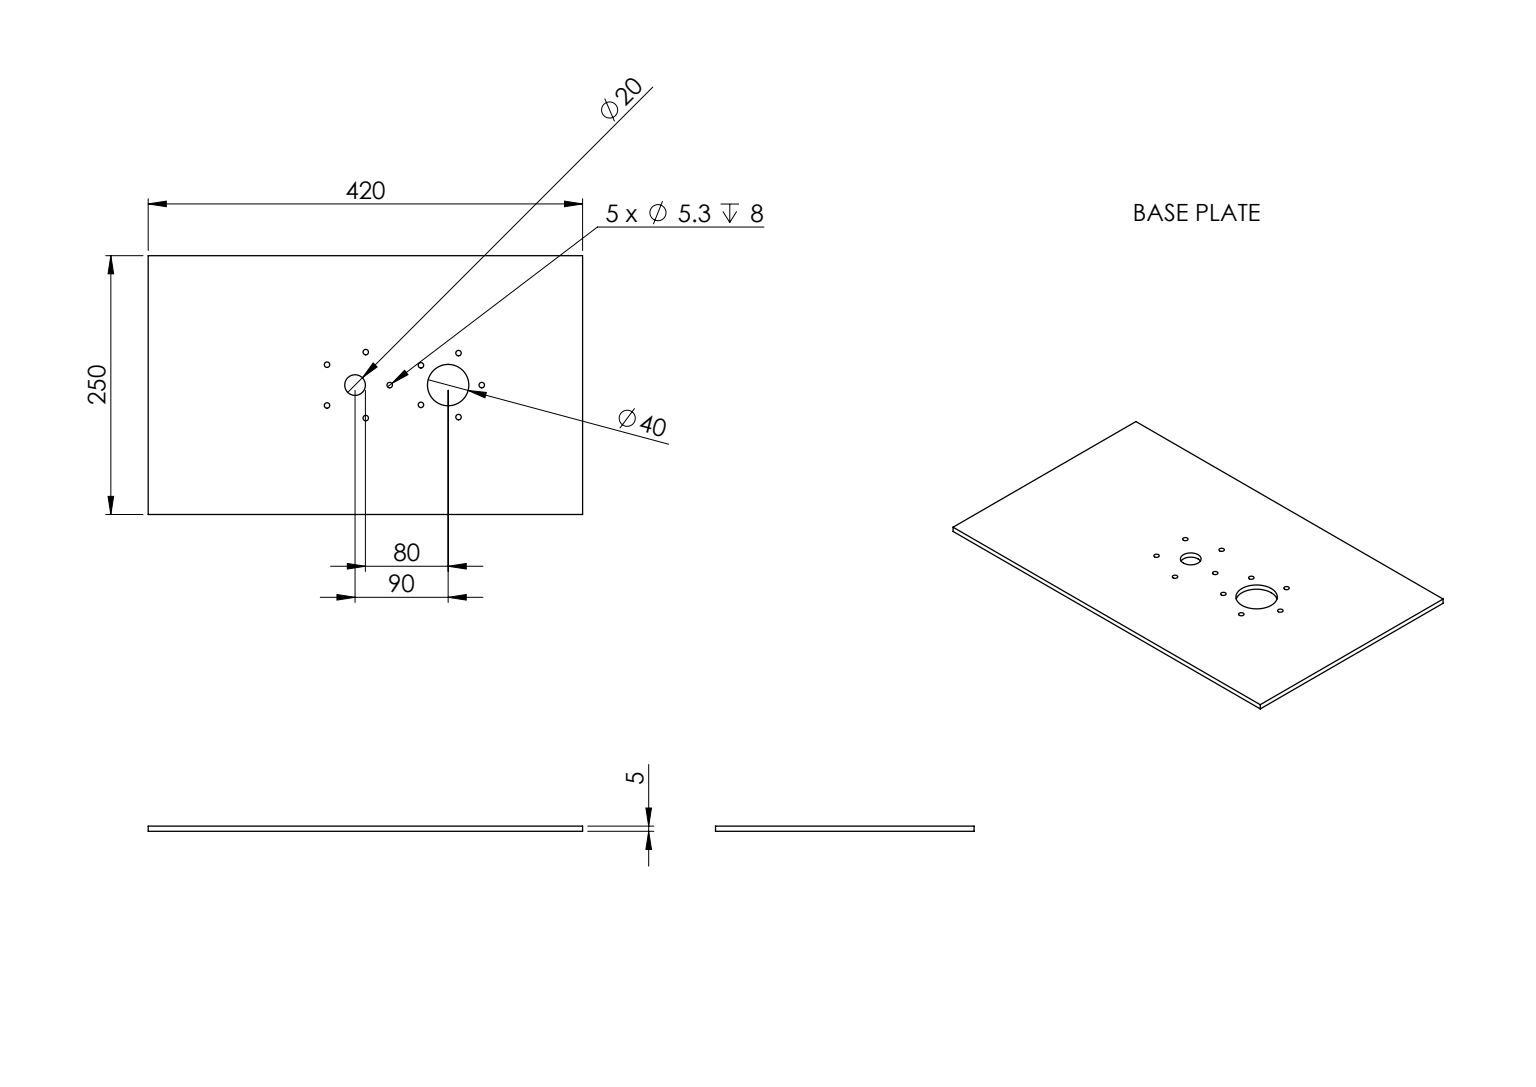
ISO-10303-21;
HEADER;
FILE_DESCRIPTION (('STEP AP214'),
    '1' );
FILE_NAME ('base plate.step',
    '2026-10-24T07:08:27',
    ( '' ),
    ( '' ),
    'SwSTEP 2.0',
    'SolidWorks 2026',
    '' );
FILE_SCHEMA (( 'AUTOMOTIVE_DESIGN' ));
ENDSEC;

DATA;
#6=VERTEX_POINT ( 'NONE', #17079 ) ;
#11=CARTESIAN_POINT ( 'NONE',  ( -79.64793068852898728, -30.00000000000000000, -31.86039329588756530 ) ) ;
#15=FACE_BOUND ( 'NONE', #1592, .T. ) ;
#41=EDGE_CURVE ( 'NONE', #17767, #6918, #12253, .T. ) ;
#44=EDGE_CURVE ( 'NONE', #931, #15024, #4657, .T. ) ;
#71=EDGE_CURVE ( 'NONE', #17356, #16127, #6478, .T. ) ;
#87=FACE_OUTER_BOUND ( 'NONE', #3507, .T. ) ;
#114=VERTEX_POINT ( 'NONE', #13345 ) ;
#120=CARTESIAN_POINT ( 'NONE',  ( -117.1020693116506379, -30.00000000000000000, -19.69080595179801207 ) ) ;
#126=COLOUR_RGB ( '',0.8941176470588234615, 0.8941176470588234615, 0.8941176470588234615 ) ;
#138=FACE_OUTER_BOUND ( 'NONE', #567, .T. ) ;
#139=VERTEX_POINT ( 'NONE', #10380 ) ;
#143=CARTESIAN_POINT ( 'NONE',  ( 0.000000000000000000, -34.99999999999999289, 20.00000000000000000 ) ) ;
#162=EDGE_CURVE ( 'NONE', #3115, #10632, #18771, .T. ) ;
#174=EDGE_CURVE ( 'NONE', #11247, #17285, #17354, .T. ) ;
#227=DIRECTION ( 'NONE',  ( -0.000000000000000000, 1.000000000000000000, -0.000000000000000000 ) ) ;
#242=CARTESIAN_POINT ( 'NONE',  ( 10.04305231718605285, -30.00000000000000000, -30.90933677959240811 ) ) ;
#257=DIRECTION ( 'NONE',  ( -0.000000000000000000, -1.000000000000000000, -0.000000000000000000 ) ) ;
#303=EDGE_CURVE ( 'NONE', #6749, #12292, #6178, .T. ) ;
#306=LINE ( 'NONE', #5042, #9675 ) ;
#312=ORIENTED_EDGE ( 'NONE', *, *, #6097, .T. ) ;
#348=EDGE_LOOP ( 'NONE', ( #7542, #2578 ) ) ;
#362=LINE ( 'NONE', #1882, #10479 ) ;
#365=DIRECTION ( 'NONE',  ( 2.220446049250313081E-16, 0.000000000000000000, 1.000000000000000000 ) ) ;
#372=EDGE_CURVE ( 'NONE', #3496, #11369, #16387, .T. ) ;
#379=EDGE_CURVE ( 'NONE', #3115, #12051, #15919, .T. ) ;
#386=VECTOR ( 'NONE', #8852, 1000.000000000000000 ) ;
#389=CARTESIAN_POINT ( 'NONE',  ( 10.04305231718605285, -26.50000000000000000, -30.90933677959240811 ) ) ;
#398=FILL_AREA_STYLE_COLOUR ( '', #126 ) ;
#409=CYLINDRICAL_SURFACE ( 'NONE', #7915, 2.649999999999995914 ) ;
#421=VERTEX_POINT ( 'NONE', #1046 ) ;
#422=ORIENTED_EDGE ( 'NONE', *, *, #16105, .T. ) ;
#425=DIRECTION ( 'NONE',  ( 0.000000000000000000, 1.000000000000000000, 0.000000000000000000 ) ) ;
#460=CARTESIAN_POINT ( 'NONE',  ( 10.04305231718579705, -30.00000000000000000, 33.55933677959249195 ) ) ;
#481=CARTESIAN_POINT ( 'NONE',  ( -79.64793068852898728, -30.00000000000000000, -31.86039329588756530 ) ) ;
#495=ORIENTED_EDGE ( 'NONE', *, *, #4462, .F. ) ;
#518=EDGE_CURVE ( 'NONE', #10933, #833, #10392, .T. ) ;
#526=ORIENTED_EDGE ( 'NONE', *, *, #16492, .F. ) ;
#533=CARTESIAN_POINT ( 'NONE',  ( 129.9999999999999432, -34.99999999999999289, -125.0000000000000000 ) ) ;
#543=DIRECTION ( 'NONE',  ( 0.000000000000000000, 0.000000000000000000, -1.000000000000000000 ) ) ;
#546=ORIENTED_EDGE ( 'NONE', *, *, #4687, .T. ) ;
#567=EDGE_LOOP ( 'NONE', ( #6055, #18455, #17783, #6474 ) ) ;
#578=EDGE_CURVE ( 'NONE', #13109, #8902, #3719, .T. ) ;
#589=DIRECTION ( 'NONE',  ( 1.000000000000000000, 0.000000000000000000, 0.000000000000000000 ) ) ;
#591=ORIENTED_EDGE ( 'NONE', *, *, #16105, .F. ) ;
#600=CARTESIAN_POINT ( 'NONE',  ( -56.50000000009000445, -34.99999999999999289, 3.817814120399276590E-13 ) ) ;
#672=FACE_OUTER_BOUND ( 'NONE', #6327, .T. ) ;
#682=PRESENTATION_STYLE_ASSIGNMENT (( #9797 ) ) ;
#690=ORIENTED_EDGE ( 'NONE', *, *, #12876, .F. ) ;
#705=EDGE_CURVE ( 'NONE', #15024, #931, #15786, .T. ) ;
#720=CARTESIAN_POINT ( 'NONE',  ( 0.000000000000000000, -34.99999999999999289, 0.000000000000000000 ) ) ;
#766=ORIENTED_EDGE ( 'NONE', *, *, #14475, .F. ) ;
#768=ORIENTED_EDGE ( 'NONE', *, *, #17161, .T. ) ;
#801=ORIENTED_EDGE ( 'NONE', *, *, #4462, .T. ) ;
#809=CIRCLE ( 'NONE', #5971, 2.649999999999999467 ) ;
#813=ORIENTED_EDGE ( 'NONE', *, *, #41, .F. ) ;
#814=CIRCLE ( 'NONE', #9625, 10.00000000000000888 ) ;
#818=FACE_BOUND ( 'NONE', #15309, .T. ) ;
#833=VERTEX_POINT ( 'NONE', #8602 ) ;
#834=ORIENTED_EDGE ( 'NONE', *, *, #10294, .F. ) ;
#842=CARTESIAN_POINT ( 'NONE',  ( -290.0000000000001137, -34.99999999999999289, -125.0000000000000000 ) ) ;
#884=ORIENTED_EDGE ( 'NONE', *, *, #8191, .T. ) ;
#891=VECTOR ( 'NONE', #1458, 1000.000000000000000 ) ;
#917=EDGE_CURVE ( 'NONE', #6918, #17767, #10543, .T. ) ;
#931=VERTEX_POINT ( 'NONE', #2514 ) ;
#992=ORIENTED_EDGE ( 'NONE', *, *, #12234, .T. ) ;
#1000=ORIENTED_EDGE ( 'NONE', *, *, #7256, .T. ) ;
#1005=DIRECTION ( 'NONE',  ( 0.000000000000000000, 0.000000000000000000, 1.000000000000000000 ) ) ;
#1046=CARTESIAN_POINT ( 'NONE',  ( -79.64793068852927149, -34.99999999999999289, 29.21039329588765554 ) ) ;
#1051=CARTESIAN_POINT ( 'NONE',  ( -117.1020693116508085, -34.99999999999999289, 19.69080595179778115 ) ) ;
#1087=CARTESIAN_POINT ( 'NONE',  ( -90.00000000009001155, -34.99999999999999289, -1.301042606982605321E-15 ) ) ;
#1117=ORIENTED_EDGE ( 'NONE', *, *, #2996, .T. ) ;
#1126=EDGE_LOOP ( 'NONE', ( #813, #5939 ) ) ;
#1159=CARTESIAN_POINT ( 'NONE',  ( -26.29305231718568336, -34.99999999999999289, -19.10302069950552095 ) ) ;
#1167=DIRECTION ( 'NONE',  ( 0.000000000000000000, 1.000000000000000000, 0.000000000000000000 ) ) ;
#1245=AXIS2_PLACEMENT_3D ( 'NONE', #17658, #4603, #10410 ) ;
#1248=ORIENTED_EDGE ( 'NONE', *, *, #16015, .T. ) ;
#1296=EDGE_CURVE ( 'NONE', #114, #9433, #4484, .T. ) ;
#1299=CARTESIAN_POINT ( 'NONE',  ( -26.29305231718584324, -26.50000000000000000, 19.10302069950530779 ) ) ;
#1300=ORIENTED_EDGE ( 'NONE', *, *, #11741, .F. ) ;
#1311=CARTESIAN_POINT ( 'NONE',  ( -117.1020693116506379, -30.00000000000000000, -19.69080595179801207 ) ) ;
#1319=CARTESIAN_POINT ( 'NONE',  ( -79.64793068852898728, -30.00000000000000000, -29.21039329588757383 ) ) ;
#1328=EDGE_CURVE ( 'NONE', #10185, #18475, #2082, .T. ) ;
#1405=ORIENTED_EDGE ( 'NONE', *, *, #12009, .T. ) ;
#1414=DIRECTION ( 'NONE',  ( 0.000000000000000000, 0.000000000000000000, 1.000000000000000000 ) ) ;
#1447=ADVANCED_FACE ( 'NONE', ( #16139 ), #17217, .F. ) ;
#1457=AXIS2_PLACEMENT_3D ( 'NONE', #120, #5912, #4495 ) ;
#1458=DIRECTION ( 'NONE',  ( -0.000000000000000000, -1.000000000000000000, -0.000000000000000000 ) ) ;
#1470=VECTOR ( 'NONE', #589, 1000.000000000000000 ) ;
#1476=FACE_OUTER_BOUND ( 'NONE', #11507, .T. ) ;
#1494=VECTOR ( 'NONE', #7308, 1000.000000000000000 ) ;
#1513=DIRECTION ( 'NONE',  ( -0.000000000000000000, 1.000000000000000000, -0.000000000000000000 ) ) ;
#1525=DIRECTION ( 'NONE',  ( 0.000000000000000000, -0.000000000000000000, 1.000000000000000000 ) ) ;
#1567=VERTEX_POINT ( 'NONE', #16419 ) ;
#1574=ORIENTED_EDGE ( 'NONE', *, *, #6302, .T. ) ;
#1583=CARTESIAN_POINT ( 'NONE',  ( -26.29305231718568336, -26.50000000000000000, -16.45302069950552237 ) ) ;
#1584=AXIS2_PLACEMENT_3D ( 'NONE', #11711, #17616, #5719 ) ;
#1592=EDGE_LOOP ( 'NONE', ( #11082, #13432 ) ) ;
#1593=ORIENTED_EDGE ( 'NONE', *, *, #16015, .F. ) ;
#1597=ORIENTED_EDGE ( 'NONE', *, *, #705, .F. ) ;
#1647=CARTESIAN_POINT ( 'NONE',  ( -290.0000000000001137, -34.99999999999999289, -125.0000000000000000 ) ) ;
#1654=EDGE_LOOP ( 'NONE', ( #3997, #6945 ) ) ;
#1700=DIRECTION ( 'NONE',  ( 0.000000000000000000, 1.000000000000000000, 0.000000000000000000 ) ) ;
#1701=ORIENTED_EDGE ( 'NONE', *, *, #15947, .F. ) ;
#1743=DIRECTION ( 'NONE',  ( -0.000000000000000000, -1.000000000000000000, -0.000000000000000000 ) ) ;
#1773=ORIENTED_EDGE ( 'NONE', *, *, #3966, .T. ) ;
#1779=EDGE_LOOP ( 'NONE', ( #16032, #2338, #6206, #546 ) ) ;
#1785=CYLINDRICAL_SURFACE ( 'NONE', #8196, 2.649999999999992806 ) ;
#1833=EDGE_LOOP ( 'NONE', ( #14175, #1300 ) ) ;
#1852=VECTOR ( 'NONE', #18637, 1000.000000000000000 ) ;
#1882=CARTESIAN_POINT ( 'NONE',  ( 130.0000000000000000, -34.99999999999999289, 125.0000000000000000 ) ) ;
#1910=FACE_OUTER_BOUND ( 'NONE', #10213, .T. ) ;
#1919=ADVANCED_FACE ( 'NONE', ( #10204 ), #2787, .F. ) ;
#1976=FACE_OUTER_BOUND ( 'NONE', #7216, .T. ) ;
#1988=DIRECTION ( 'NONE',  ( -0.000000000000000000, -1.000000000000000000, -0.000000000000000000 ) ) ;
#2004=DIRECTION ( 'NONE',  ( -0.000000000000000000, 1.000000000000000000, -0.000000000000000000 ) ) ;
#2019=EDGE_CURVE ( 'NONE', #5476, #6010, #306, .T. ) ;
#2034=LINE ( 'NONE', #6412, #15369 ) ;
#2063=DIRECTION ( 'NONE',  ( 0.000000000000000000, 0.000000000000000000, 1.000000000000000000 ) ) ;
#2079=ADVANCED_FACE ( 'NONE', ( #3250 ), #13448, .F. ) ;
#2082=LINE ( 'NONE', #6544, #18168 ) ;
#2096=DIRECTION ( 'NONE',  ( 0.000000000000000000, 0.000000000000000000, 1.000000000000000000 ) ) ;
#2099=ADVANCED_FACE ( 'NONE', ( #1910 ), #13533, .F. ) ;
#2102=DIRECTION ( 'NONE',  ( -0.000000000000000000, 1.000000000000000000, -0.000000000000000000 ) ) ;
#2142=DIRECTION ( 'NONE',  ( -0.000000000000000000, 1.000000000000000000, -0.000000000000000000 ) ) ;
#2144=FACE_BOUND ( 'NONE', #18626, .T. ) ;
#2188=DIRECTION ( 'NONE',  ( -0.000000000000000000, 1.000000000000000000, -0.000000000000000000 ) ) ;
#2232=ORIENTED_EDGE ( 'NONE', *, *, #12399, .T. ) ;
#2246=( GEOMETRIC_REPRESENTATION_CONTEXT ( 3 ) GLOBAL_UNCERTAINTY_ASSIGNED_CONTEXT ( ( #14139 ) ) GLOBAL_UNIT_ASSIGNED_CONTEXT ( ( #8004, #17231, #15165 ) ) REPRESENTATION_CONTEXT ( 'NONE', 'WORKASPACE' ) );
#2260=VERTEX_POINT ( 'NONE', #16093 ) ;
#2267=VERTEX_POINT ( 'NONE', #14659 ) ;
#2289=EDGE_CURVE ( 'NONE', #10632, #8217, #5434, .T. ) ;
#2299=CARTESIAN_POINT ( 'NONE',  ( -26.29305231718568336, -30.00000000000000000, -16.45302069950552237 ) ) ;
#2307=EDGE_LOOP ( 'NONE', ( #14097, #884, #7375, #8235 ) ) ;
#2310=ORIENTED_EDGE ( 'NONE', *, *, #9236, .T. ) ;
#2316=ORIENTED_EDGE ( 'NONE', *, *, #12234, .F. ) ;
#2338=ORIENTED_EDGE ( 'NONE', *, *, #11370, .F. ) ;
#2339=EDGE_LOOP ( 'NONE', ( #17775, #17142 ) ) ;
#2344=VECTOR ( 'NONE', #9583, 1000.000000000000000 ) ;
#2404=EDGE_LOOP ( 'NONE', ( #3864, #2415 ) ) ;
#2415=ORIENTED_EDGE ( 'NONE', *, *, #303, .F. ) ;
#2422=VERTEX_POINT ( 'NONE', #17894 ) ;
#2494=ADVANCED_FACE ( 'NONE', ( #11888 ), #13334, .F. ) ;
#2497=CARTESIAN_POINT ( 'NONE',  ( -290.0000000000001137, -30.00000000000000000, -125.0000000000000000 ) ) ;
#2499=CYLINDRICAL_SURFACE ( 'NONE', #10518, 2.649999999999995914 ) ;
#2514=CARTESIAN_POINT ( 'NONE',  ( -26.29305231718584324, -34.99999999999999289, 16.45302069950530566 ) ) ;
#2578=ORIENTED_EDGE ( 'NONE', *, *, #11344, .F. ) ;
#2592=CARTESIAN_POINT ( 'NONE',  ( 0.000000000000000000, -30.00000000000000000, 0.000000000000000000 ) ) ;
#2593=CARTESIAN_POINT ( 'NONE',  ( 32.50000000000000000, -34.99999999999999289, 3.680389326632394941E-13 ) ) ;
#2626=DIRECTION ( 'NONE',  ( 0.000000000000000000, 1.000000000000000000, 0.000000000000000000 ) ) ;
#2633=AXIS2_PLACEMENT_3D ( 'NONE', #6245, #17768, #15017 ) ;
#2671=LINE ( 'NONE', #10001, #13888 ) ;
#2678=CARTESIAN_POINT ( 'NONE',  ( -90.00000000009001155, -29.99899999999999878, -1.301042606982605321E-15 ) ) ;
#2679=VECTOR ( 'NONE', #12131, 1000.000000000000000 ) ;
#2705=PRODUCT_CONTEXT ( 'NONE', #4283, 'mechanical' ) ;
#2757=DIRECTION ( 'NONE',  ( 0.000000000000000000, 0.000000000000000000, 1.000000000000000000 ) ) ;
#2770=DIRECTION ( 'NONE',  ( 0.000000000000000000, 1.000000000000000000, 0.000000000000000000 ) ) ;
#2773=STYLED_ITEM('',(#18855),#10108);
#2783=DIRECTION ( 'NONE',  ( -1.000000000000000000, 0.000000000000000000, -0.000000000000000000 ) ) ;
#2787=CYLINDRICAL_SURFACE ( 'NONE', #1457, 2.649999999999992806 ) ;
#2827=EDGE_CURVE ( 'NONE', #16722, #5310, #4082, .T. ) ;
#2846=ADVANCED_FACE ( 'NONE', ( #17872 ), #16535, .F. ) ;
#2854=CARTESIAN_POINT ( 'NONE',  ( -117.1020693116508085, -30.00000000000000000, 22.34080595179776907 ) ) ;
#2864=CARTESIAN_POINT ( 'NONE',  ( 2.449293598294706513E-15, -34.99999999999999289, -20.00000000000000000 ) ) ;
#2868=CARTESIAN_POINT ( 'NONE',  ( 129.9999999999999432, -34.99999999999999289, -125.0000000000000000 ) ) ;
#2885=DIRECTION ( 'NONE',  ( -0.000000000000000000, 1.000000000000000000, -0.000000000000000000 ) ) ;
#2888=ORIENTED_EDGE ( 'NONE', *, *, #17161, .F. ) ;
#2954=EDGE_CURVE ( 'NONE', #3496, #10145, #7497, .T. ) ;
#2979=CIRCLE ( 'NONE', #14535, 2.649999999999995914 ) ;
#2996=EDGE_CURVE ( 'NONE', #15825, #6010, #809, .T. ) ;
#3009=CYLINDRICAL_SURFACE ( 'NONE', #15827, 2.649999999999999467 ) ;
#3019=CARTESIAN_POINT ( 'NONE',  ( 10.04305231718579705, -26.50000000000000000, 28.25933677959249835 ) ) ;
#3089=DIRECTION ( 'NONE',  ( 0.000000000000000000, 0.000000000000000000, 1.000000000000000000 ) ) ;
#3115=VERTEX_POINT ( 'NONE', #3969 ) ;
#3156=DIRECTION ( 'NONE',  ( -0.000000000000000000, 1.000000000000000000, -0.000000000000000000 ) ) ;
#3161=( GEOMETRIC_REPRESENTATION_CONTEXT ( 3 ) GLOBAL_UNCERTAINTY_ASSIGNED_CONTEXT ( ( #15290 ) ) GLOBAL_UNIT_ASSIGNED_CONTEXT ( ( #14683, #18007, #11919 ) ) REPRESENTATION_CONTEXT ( 'NONE', 'WORKASPACE' ) );
#3175=CARTESIAN_POINT ( 'NONE',  ( -56.50000000009000445, -30.00000000000000000, 3.817814120399276590E-13 ) ) ;
#3197=CARTESIAN_POINT ( 'NONE',  ( -117.1020693116506379, -30.00000000000000000, -22.34080595179799644 ) ) ;
#3218=VECTOR ( 'NONE', #2004, 1000.000000000000000 ) ;
#3222=ORIENTED_EDGE ( 'NONE', *, *, #2827, .T. ) ;
#3230=DIRECTION ( 'NONE',  ( 0.000000000000000000, 0.000000000000000000, 1.000000000000000000 ) ) ;
#3233=FACE_BOUND ( 'NONE', #18034, .T. ) ;
#3237=ORIENTED_EDGE ( 'NONE', *, *, #518, .T. ) ;
#3250=FACE_OUTER_BOUND ( 'NONE', #18743, .T. ) ;
#3293=PRODUCT ( 'base plate', 'base plate', '', ( #2705 ) ) ;
#3320=AXIS2_PLACEMENT_3D ( 'NONE', #12306, #11167, #13832 ) ;
#3345=CARTESIAN_POINT ( 'NONE',  ( 32.50000000000000000, -26.50000000000000000, 2.650000000000367617 ) ) ;
#3388=CYLINDRICAL_SURFACE ( 'NONE', #15829, 2.649999999999999467 ) ;
#3415=CYLINDRICAL_SURFACE ( 'NONE', #15730, 2.649999999999992806 ) ;
#3430=DIRECTION ( 'NONE',  ( 0.000000000000000000, 0.000000000000000000, 1.000000000000000000 ) ) ;
#3433=EDGE_CURVE ( 'NONE', #12463, #15108, #11438, .T. ) ;
#3451=ORIENTED_EDGE ( 'NONE', *, *, #4742, .F. ) ;
#3461=DIRECTION ( 'NONE',  ( -0.000000000000000000, 1.000000000000000000, -0.000000000000000000 ) ) ;
#3465=CYLINDRICAL_SURFACE ( 'NONE', #14086, 2.649999999999992806 ) ;
#3490=CARTESIAN_POINT ( 'NONE',  ( -90.00000000009001155, -29.99899999999999878, -1.301042606982605321E-15 ) ) ;
#3496=VERTEX_POINT ( 'NONE', #18587 ) ;
#3507=EDGE_LOOP ( 'NONE', ( #14888, #591, #4877, #1000 ) ) ;
#3509=DIRECTION ( 'NONE',  ( -0.000000000000000000, 1.000000000000000000, -0.000000000000000000 ) ) ;
#3513=ADVANCED_FACE ( 'NONE', ( #9908 ), #15727, .F. ) ;
#3530=AXIS2_PLACEMENT_3D ( 'NONE', #15724, #12775, #17155 ) ;
#3559=AXIS2_PLACEMENT_3D ( 'NONE', #6389, #10947, #13724 ) ;
#3582=AXIS2_PLACEMENT_3D ( 'NONE', #8174, #9587, #15407 ) ;
#3584=FACE_OUTER_BOUND ( 'NONE', #16769, .T. ) ;
#3589=VERTEX_POINT ( 'NONE', #2864 ) ;
#3611=CARTESIAN_POINT ( 'NONE',  ( -79.64793068852898728, -30.00000000000000000, -29.21039329588758093 ) ) ;
#3659=VERTEX_POINT ( 'NONE', #6466 ) ;
#3679=EDGE_LOOP ( 'NONE', ( #8260, #18538, #18212, #10633 ) ) ;
#3692=DIRECTION ( 'NONE',  ( -0.000000000000000000, 1.000000000000000000, -0.000000000000000000 ) ) ;
#3719=CIRCLE ( 'NONE', #6141, 2.649999999999995914 ) ;
#3740=CARTESIAN_POINT ( 'NONE',  ( 10.04305231718579705, -34.99999999999999289, 28.25933677959249835 ) ) ;
#3745=ORIENTED_EDGE ( 'NONE', *, *, #162, .T. ) ;
#3763=PLANE ( 'NONE',  #9122 ) ;
#3771=CARTESIAN_POINT ( 'NONE',  ( -26.29305231718568336, -30.00000000000000000, -19.10302069950552095 ) ) ;
#3780=DIRECTION ( 'NONE',  ( 0.000000000000000000, 0.000000000000000000, 1.000000000000000000 ) ) ;
#3806=ORIENTED_EDGE ( 'NONE', *, *, #11750, .F. ) ;
#3864=ORIENTED_EDGE ( 'NONE', *, *, #17557, .F. ) ;
#3885=AXIS2_PLACEMENT_3D ( 'NONE', #17001, #3954, #5176 ) ;
#3900=ORIENTED_EDGE ( 'NONE', *, *, #18325, .T. ) ;
#3931=DIRECTION ( 'NONE',  ( -0.000000000000000000, -1.000000000000000000, -0.000000000000000000 ) ) ;
#3945=VECTOR ( 'NONE', #14406, 1000.000000000000000 ) ;
#3954=DIRECTION ( 'NONE',  ( -0.000000000000000000, 0.000000000000000000, 1.000000000000000000 ) ) ;
#3966=EDGE_CURVE ( 'NONE', #16722, #9159, #4728, .T. ) ;
#3968=ORIENTED_EDGE ( 'NONE', *, *, #2019, .F. ) ;
#3969=CARTESIAN_POINT ( 'NONE',  ( -90.00000000009001155, -30.00000000000000000, 10.00000000000000711 ) ) ;
#3982=LINE ( 'NONE', #18447, #1852 ) ;
#3997=ORIENTED_EDGE ( 'NONE', *, *, #10814, .F. ) ;
#4006=ORIENTED_EDGE ( 'NONE', *, *, #16784, .F. ) ;
#4022=DIRECTION ( 'NONE',  ( 0.000000000000000000, 0.000000000000000000, 1.000000000000000000 ) ) ;
#4056=CARTESIAN_POINT ( 'NONE',  ( -117.1020693116506379, -34.99999999999999289, -17.04080595179801705 ) ) ;
#4072=CARTESIAN_POINT ( 'NONE',  ( 10.04305231718605285, -26.50000000000000000, -33.55933677959240669 ) ) ;
#4073=EDGE_LOOP ( 'NONE', ( #11865, #9142, #15557, #1248 ) ) ;
#4076=DIRECTION ( 'NONE',  ( -0.000000000000000000, 1.000000000000000000, -0.000000000000000000 ) ) ;
#4080=CARTESIAN_POINT ( 'NONE',  ( 0.000000000000000000, -34.99999999999999289, 0.000000000000000000 ) ) ;
#4082=LINE ( 'NONE', #1319, #1494 ) ;
#4109=DIRECTION ( 'NONE',  ( 0.000000000000000000, 0.000000000000000000, 1.000000000000000000 ) ) ;
#4179=AXIS2_PLACEMENT_3D ( 'NONE', #18479, #12480, #18285 ) ;
#4191=VECTOR ( 'NONE', #16551, 1000.000000000000000 ) ;
#4283=APPLICATION_CONTEXT ( 'automotive_design' ) ;
#4303=EDGE_CURVE ( 'NONE', #2260, #2267, #7470, .T. ) ;
#4306=ORIENTED_EDGE ( 'NONE', *, *, #1296, .F. ) ;
#4321=CARTESIAN_POINT ( 'NONE',  ( -79.64793068852898728, -30.00000000000000000, -34.51039329588756033 ) ) ;
#4325=CIRCLE ( 'NONE', #15894, 2.649999999999999467 ) ;
#4392=FACE_OUTER_BOUND ( 'NONE', #4549, .T. ) ;
#4395=CARTESIAN_POINT ( 'NONE',  ( 129.9999999999999432, -34.99999999999999289, -125.0000000000000000 ) ) ;
#4421=CARTESIAN_POINT ( 'NONE',  ( 0.000000000000000000, -34.99999999999999289, 0.000000000000000000 ) ) ;
#4425=ORIENTED_EDGE ( 'NONE', *, *, #4303, .T. ) ;
#4446=ORIENTED_EDGE ( 'NONE', *, *, #17557, .T. ) ;
#4462=EDGE_CURVE ( 'NONE', #17285, #14160, #6227, .T. ) ;
#4468=EDGE_LOOP ( 'NONE', ( #17730, #15846 ) ) ;
#4484=CIRCLE ( 'NONE', #3582, 2.649999999999995914 ) ;
#4495=DIRECTION ( 'NONE',  ( 0.000000000000000000, 0.000000000000000000, 1.000000000000000000 ) ) ;
#4509=VECTOR ( 'NONE', #10191, 1000.000000000000000 ) ;
#4549=EDGE_LOOP ( 'NONE', ( #992, #4614, #495, #17288 ) ) ;
#4551=FACE_OUTER_BOUND ( 'NONE', #17127, .T. ) ;
#4563=FACE_BOUND ( 'NONE', #1833, .T. ) ;
#4586=CARTESIAN_POINT ( 'NONE',  ( -26.29305231718584324, -26.50000000000000000, 21.75302069950530637 ) ) ;
#4603=DIRECTION ( 'NONE',  ( -0.000000000000000000, 1.000000000000000000, -0.000000000000000000 ) ) ;
#4605=DIRECTION ( 'NONE',  ( -0.000000000000000000, 1.000000000000000000, -0.000000000000000000 ) ) ;
#4606=DIRECTION ( 'NONE',  ( 0.000000000000000000, -1.000000000000000000, 0.000000000000000000 ) ) ;
#4614=ORIENTED_EDGE ( 'NONE', *, *, #7486, .F. ) ;
#4639=ORIENTED_EDGE ( 'NONE', *, *, #15062, .T. ) ;
#4657=CIRCLE ( 'NONE', #7088, 2.649999999999999467 ) ;
#4687=EDGE_CURVE ( 'NONE', #8217, #10632, #814, .T. ) ;
#4690=DIRECTION ( 'NONE',  ( 0.000000000000000000, 0.000000000000000000, 1.000000000000000000 ) ) ;
#4726=EDGE_LOOP ( 'NONE', ( #3806, #16728, #16453, #2316 ) ) ;
#4727=CARTESIAN_POINT ( 'NONE',  ( -117.1020693116508085, -30.00000000000000000, 19.69080595179778115 ) ) ;
#4728=CIRCLE ( 'NONE', #15680, 2.649999999999992806 ) ;
#4736=CARTESIAN_POINT ( 'NONE',  ( -117.1020693116508085, -30.00000000000000000, 19.69080595179778115 ) ) ;
#4742=EDGE_CURVE ( 'NONE', #421, #6727, #6673, .T. ) ;
#4762=ADVANCED_FACE ( 'NONE', ( #672 ), #6759, .F. ) ;
#4764=EDGE_LOOP ( 'NONE', ( #17958, #10734 ) ) ;
#4815=DIRECTION ( 'NONE',  ( -1.000000000000000000, 0.000000000000000000, 2.220446049250313081E-16 ) ) ;
#4827=ORIENTED_EDGE ( 'NONE', *, *, #372, .T. ) ;
#4877=ORIENTED_EDGE ( 'NONE', *, *, #12760, .T. ) ;
#4887=DIRECTION ( 'NONE',  ( -0.000000000000000000, 1.000000000000000000, -0.000000000000000000 ) ) ;
#4929=ORIENTED_EDGE ( 'NONE', *, *, #16784, .T. ) ;
#4948=AXIS2_PLACEMENT_3D ( 'NONE', #2592, #5353, #9643 ) ;
#4985=EDGE_LOOP ( 'NONE', ( #4306, #5955 ) ) ;
#4989=FACE_OUTER_BOUND ( 'NONE', #4073, .T. ) ;
#5012=DIRECTION ( 'NONE',  ( 0.000000000000000000, 0.000000000000000000, 1.000000000000000000 ) ) ;
#5015=LINE ( 'NONE', #18072, #16336 ) ;
#5019=CARTESIAN_POINT ( 'NONE',  ( 10.04305231718605285, -30.00000000000000000, -33.55933677959240669 ) ) ;
#5024=DIRECTION ( 'NONE',  ( 0.000000000000000000, 1.000000000000000000, 0.000000000000000000 ) ) ;
#5028=ADVANCED_FACE ( 'NONE', ( #16462 ), #3415, .F. ) ;
#5035=ORIENTED_EDGE ( 'NONE', *, *, #16675, .F. ) ;
#5042=CARTESIAN_POINT ( 'NONE',  ( -26.29305231718568336, -26.50000000000000000, -21.75302069950551953 ) ) ;
#5045=CARTESIAN_POINT ( 'NONE',  ( -26.29305231718584324, -30.00000000000000000, 16.45302069950530566 ) ) ;
#5065=FACE_OUTER_BOUND ( 'NONE', #11763, .T. ) ;
#5075=ORIENTED_EDGE ( 'NONE', *, *, #379, .T. ) ;
#5090=FACE_BOUND ( 'NONE', #4468, .T. ) ;
#5119=DIRECTION ( 'NONE',  ( 0.000000000000000000, 0.000000000000000000, 1.000000000000000000 ) ) ;
#5122=CARTESIAN_POINT ( 'NONE',  ( -56.50000000009000445, -30.00000000000000000, 3.817814120399276590E-13 ) ) ;
#5159=LINE ( 'NONE', #9635, #11465 ) ;
#5160=CARTESIAN_POINT ( 'NONE',  ( 10.04305231718605285, -26.50000000000000000, -30.90933677959240811 ) ) ;
#5176=DIRECTION ( 'NONE',  ( 1.000000000000000000, 0.000000000000000000, 0.000000000000000000 ) ) ;
#5198=EDGE_LOOP ( 'NONE', ( #3451, #690, #8535, #5749 ) ) ;
#5242=CARTESIAN_POINT ( 'NONE',  ( 10.04305231718579705, -30.00000000000000000, 30.90933677959249337 ) ) ;
#5259=EDGE_LOOP ( 'NONE', ( #17923, #5075 ) ) ;
#5310=VERTEX_POINT ( 'NONE', #3611 ) ;
#5335=DIRECTION ( 'NONE',  ( 0.000000000000000000, 0.000000000000000000, 1.000000000000000000 ) ) ;
#5353=DIRECTION ( 'NONE',  ( 0.000000000000000000, -1.000000000000000000, 0.000000000000000000 ) ) ;
#5406=( NAMED_UNIT ( * ) SI_UNIT ( $, .STERADIAN. ) SOLID_ANGLE_UNIT ( ) );
#5417=ADVANCED_FACE ( 'NONE', ( #1976 ), #6080, .F. ) ;
#5434=CIRCLE ( 'NONE', #16368, 10.00000000000000888 ) ;
#5446=CYLINDRICAL_SURFACE ( 'NONE', #3530, 2.649999999999995914 ) ;
#5476=VERTEX_POINT ( 'NONE', #18453 ) ;
#5477=DIRECTION ( 'NONE',  ( 0.000000000000000000, 0.000000000000000000, -1.000000000000000000 ) ) ;
#5488=DIRECTION ( 'NONE',  ( -0.000000000000000000, -1.000000000000000000, -0.000000000000000000 ) ) ;
#5535=CIRCLE ( 'NONE', #1245, 2.649999999999985700 ) ;
#5609=CARTESIAN_POINT ( 'NONE',  ( 130.0000000000000000, -34.99999999999999289, 125.0000000000000000 ) ) ;
#5638=VERTEX_POINT ( 'NONE', #8459 ) ;
#5681=CIRCLE ( 'NONE', #9629, 10.00000000000000888 ) ;
#5701=ORIENTED_EDGE ( 'NONE', *, *, #705, .T. ) ;
#5719=DIRECTION ( 'NONE',  ( 0.000000000000000000, 0.000000000000000000, 1.000000000000000000 ) ) ;
#5729=CIRCLE ( 'NONE', #12952, 2.649999999999985700 ) ;
#5735=CARTESIAN_POINT ( 'NONE',  ( 2.449293598294706513E-15, -34.99999999999999289, -20.00000000000000000 ) ) ;
#5749=ORIENTED_EDGE ( 'NONE', *, *, #15654, .T. ) ;
#5767=AXIS2_PLACEMENT_3D ( 'NONE', #10264, #10359, #5798 ) ;
#5780=AXIS2_PLACEMENT_3D ( 'NONE', #15587, #10875, #8121 ) ;
#5787=PRODUCT_DEFINITION_CONTEXT ( 'detailed design', #16821, 'design' ) ;
#5798=DIRECTION ( 'NONE',  ( 0.000000000000000000, 0.000000000000000000, 1.000000000000000000 ) ) ;
#5807=DIRECTION ( 'NONE',  ( -0.000000000000000000, 1.000000000000000000, -0.000000000000000000 ) ) ;
#5809=DIRECTION ( 'NONE',  ( 0.000000000000000000, 0.000000000000000000, -1.000000000000000000 ) ) ;
#5811=FACE_BOUND ( 'NONE', #13280, .T. ) ;
#5820=ORIENTED_EDGE ( 'NONE', *, *, #7851, .T. ) ;
#5912=DIRECTION ( 'NONE',  ( -0.000000000000000000, 1.000000000000000000, -0.000000000000000000 ) ) ;
#5939=ORIENTED_EDGE ( 'NONE', *, *, #917, .F. ) ;
#5948=AXIS2_PLACEMENT_3D ( 'NONE', #8035, #2142, #1005 ) ;
#5955=ORIENTED_EDGE ( 'NONE', *, *, #7794, .F. ) ;
#5966=DIRECTION ( 'NONE',  ( 0.000000000000000000, 1.000000000000000000, 0.000000000000000000 ) ) ;
#5971=AXIS2_PLACEMENT_3D ( 'NONE', #3771, #15211, #2063 ) ;
#5973=CARTESIAN_POINT ( 'NONE',  ( -117.1020693116508085, -30.00000000000000000, 17.04080595179779678 ) ) ;
#6010=VERTEX_POINT ( 'NONE', #13005 ) ;
#6041=CIRCLE ( 'NONE', #14569, 2.649999999999992806 ) ;
#6055=ORIENTED_EDGE ( 'NONE', *, *, #9841, .T. ) ;
#6080=CYLINDRICAL_SURFACE ( 'NONE', #13302, 2.649999999999999467 ) ;
#6092=CARTESIAN_POINT ( 'NONE',  ( -90.00000000009001155, -29.99899999999999878, 10.00000000000000711 ) ) ;
#6097=EDGE_CURVE ( 'NONE', #833, #10933, #8182, .T. ) ;
#6100=DIRECTION ( 'NONE',  ( 0.000000000000000000, 0.000000000000000000, -1.000000000000000000 ) ) ;
#6120=ORIENTED_EDGE ( 'NONE', *, *, #303, .T. ) ;
#6129=EDGE_LOOP ( 'NONE', ( #5701, #11141, #6120, #9815 ) ) ;
#6141=AXIS2_PLACEMENT_3D ( 'NONE', #242, #425, #2757 ) ;
#6146=LINE ( 'NONE', #13204, #7038 ) ;
#6163=VECTOR ( 'NONE', #8667, 1000.000000000000000 ) ;
#6173=CIRCLE ( 'NONE', #9227, 20.00000000000000000 ) ;
#6178=CIRCLE ( 'NONE', #16833, 2.649999999999999467 ) ;
#6194=DIRECTION ( 'NONE',  ( -0.000000000000000000, 1.000000000000000000, -0.000000000000000000 ) ) ;
#6195=CARTESIAN_POINT ( 'NONE',  ( -117.1020693116506379, -30.00000000000000000, -22.34080595179800355 ) ) ;
#6206=ORIENTED_EDGE ( 'NONE', *, *, #6438, .T. ) ;
#6215=ADVANCED_FACE ( 'NONE', ( #138 ), #10691, .F. ) ;
#6227=LINE ( 'NONE', #9178, #13878 ) ;
#6245=CARTESIAN_POINT ( 'NONE',  ( 32.50000000000000000, -34.99999999999999289, 3.680389326632394941E-13 ) ) ;
#6290=DIRECTION ( 'NONE',  ( -0.000000000000000000, 1.000000000000000000, -0.000000000000000000 ) ) ;
#6291=LINE ( 'NONE', #6195, #17102 ) ;
#6302=EDGE_CURVE ( 'NONE', #421, #10185, #9579, .T. ) ;
#6327=EDGE_LOOP ( 'NONE', ( #13120, #2232, #4827, #6580 ) ) ;
#6332=ORIENTED_EDGE ( 'NONE', *, *, #10747, .T. ) ;
#6340=FACE_BOUND ( 'NONE', #7111, .T. ) ;
#6359=AXIS2_PLACEMENT_3D ( 'NONE', #8802, #5488, #15365 ) ;
#6389=CARTESIAN_POINT ( 'NONE',  ( 32.50000000000000000, -30.00000000000000000, 3.680389326632394941E-13 ) ) ;
#6412=CARTESIAN_POINT ( 'NONE',  ( -290.0000000000001705, -30.00000000000000000, 125.0000000000000000 ) ) ;
#6422=AXIS2_PLACEMENT_3D ( 'NONE', #13352, #6100, #2783 ) ;
#6432=VECTOR ( 'NONE', #14818, 1000.000000000000000 ) ;
#6438=EDGE_CURVE ( 'NONE', #12051, #8217, #10030, .T. ) ;
#6466=CARTESIAN_POINT ( 'NONE',  ( -117.1020693116506379, -30.00000000000000000, -17.04080595179802415 ) ) ;
#6474=ORIENTED_EDGE ( 'NONE', *, *, #7486, .T. ) ;
#6478=CIRCLE ( 'NONE', #9514, 2.649999999999985700 ) ;
#6484=ORIENTED_EDGE ( 'NONE', *, *, #41, .T. ) ;
#6542=EDGE_CURVE ( 'NONE', #2260, #17356, #15748, .T. ) ;
#6544=CARTESIAN_POINT ( 'NONE',  ( -79.64793068852927149, -30.00000000000000000, 34.51039329588763849 ) ) ;
#6553=ORIENTED_EDGE ( 'NONE', *, *, #14839, .T. ) ;
#6580=ORIENTED_EDGE ( 'NONE', *, *, #13036, .T. ) ;
#6587=VECTOR ( 'NONE', #15638, 1000.000000000000000 ) ;
#6590=EDGE_LOOP ( 'NONE', ( #422, #4425 ) ) ;
#6597=CYLINDRICAL_SURFACE ( 'NONE', #12972, 2.649999999999999467 ) ;
#6622=FACE_BOUND ( 'NONE', #4764, .T. ) ;
#6671=AXIS2_PLACEMENT_3D ( 'NONE', #12341, #3692, #3780 ) ;
#6673=LINE ( 'NONE', #14090, #17257 ) ;
#6676=CYLINDRICAL_SURFACE ( 'NONE', #4179, 2.649999999999999467 ) ;
#6727=VERTEX_POINT ( 'NONE', #16491 ) ;
#6749=VERTEX_POINT ( 'NONE', #5045 ) ;
#6759=CYLINDRICAL_SURFACE ( 'NONE', #18149, 2.649999999999999467 ) ;
#6800=DIRECTION ( 'NONE',  ( 0.000000000000000000, 0.000000000000000000, 1.000000000000000000 ) ) ;
#6804=FACE_OUTER_BOUND ( 'NONE', #7060, .T. ) ;
#6816=ORIENTED_EDGE ( 'NONE', *, *, #8524, .F. ) ;
#6823=ORIENTED_EDGE ( 'NONE', *, *, #12399, .F. ) ;
#6841=CARTESIAN_POINT ( 'NONE',  ( 10.04305231718579705, -34.99999999999999289, 30.90933677959249337 ) ) ;
#6858=CARTESIAN_POINT ( 'NONE',  ( 10.04305231718579705, -30.00000000000000000, 28.25933677959249835 ) ) ;
#6901=AXIS2_PLACEMENT_3D ( 'NONE', #7078, #12709, #6800 ) ;
#6918=VERTEX_POINT ( 'NONE', #6858 ) ;
#6932=ORIENTED_EDGE ( 'NONE', *, *, #13644, .F. ) ;
#6945=ORIENTED_EDGE ( 'NONE', *, *, #17454, .F. ) ;
#7026=ORIENTED_EDGE ( 'NONE', *, *, #9236, .F. ) ;
#7038=VECTOR ( 'NONE', #10622, 1000.000000000000000 ) ;
#7060=EDGE_LOOP ( 'NONE', ( #526, #768, #17611, #1701 ) ) ;
#7076=SHAPE_DEFINITION_REPRESENTATION ( #9060, #18682 ) ;
#7078=CARTESIAN_POINT ( 'NONE',  ( 10.04305231718579705, -30.00000000000000000, 30.90933677959249337 ) ) ;
#7088=AXIS2_PLACEMENT_3D ( 'NONE', #15632, #3931, #4109 ) ;
#7100=DIRECTION ( 'NONE',  ( -0.000000000000000000, 1.000000000000000000, -0.000000000000000000 ) ) ;
#7102=CARTESIAN_POINT ( 'NONE',  ( -79.64793068852927149, -34.99999999999999289, 34.51039329588763849 ) ) ;
#7111=EDGE_LOOP ( 'NONE', ( #1597, #8219 ) ) ;
#7112=ORIENTED_EDGE ( 'NONE', *, *, #15654, .F. ) ;
#7114=SURFACE_STYLE_FILL_AREA ( #9437 ) ;
#7201=ORIENTED_EDGE ( 'NONE', *, *, #12482, .T. ) ;
#7216=EDGE_LOOP ( 'NONE', ( #3968, #9071, #15983, #1117 ) ) ;
#7229=CYLINDRICAL_SURFACE ( 'NONE', #12694, 2.649999999999992806 ) ;
#7232=CARTESIAN_POINT ( 'NONE',  ( -56.50000000009000445, -30.00000000000000000, 3.817814120399276590E-13 ) ) ;
#7240=CARTESIAN_POINT ( 'NONE',  ( -90.00000000009001155, -34.99999999999999289, -10.00000000000001066 ) ) ;
#7243=AXIS2_PLACEMENT_3D ( 'NONE', #481, #12671, #10948 ) ;
#7256=EDGE_CURVE ( 'NONE', #16127, #17356, #14913, .T. ) ;
#7290=ADVANCED_FACE ( 'NONE', ( #14618 ), #3009, .F. ) ;
#7308=DIRECTION ( 'NONE',  ( -0.000000000000000000, 1.000000000000000000, -0.000000000000000000 ) ) ;
#7310=ORIENTED_EDGE ( 'NONE', *, *, #6438, .F. ) ;
#7375=ORIENTED_EDGE ( 'NONE', *, *, #11344, .T. ) ;
#7385=AXIS2_PLACEMENT_3D ( 'NONE', #5242, #1167, #4022 ) ;
#7415=PLANE ( 'NONE',  #13584 ) ;
#7451=CYLINDRICAL_SURFACE ( 'NONE', #9434, 2.649999999999992806 ) ;
#7470=CIRCLE ( 'NONE', #18736, 2.649999999999992806 ) ;
#7477=AXIS2_PLACEMENT_3D ( 'NONE', #14747, #1700, #7514 ) ;
#7486=EDGE_CURVE ( 'NONE', #14160, #17232, #16145, .T. ) ;
#7488=CARTESIAN_POINT ( 'NONE',  ( 0.000000000000000000, -30.00000000000000000, 0.000000000000000000 ) ) ;
#7497=CIRCLE ( 'NONE', #2633, 2.649999999999999467 ) ;
#7514=DIRECTION ( 'NONE',  ( 0.000000000000000000, 0.000000000000000000, 1.000000000000000000 ) ) ;
#7521=EDGE_CURVE ( 'NONE', #114, #8902, #11853, .T. ) ;
#7523=AXIS2_PLACEMENT_3D ( 'NONE', #1311, #7100, #12923 ) ;
#7524=AXIS2_PLACEMENT_3D ( 'NONE', #16042, #4076, #9875 ) ;
#7527=PLANE ( 'NONE',  #6422 ) ;
#7529=ORIENTED_EDGE ( 'NONE', *, *, #518, .F. ) ;
#7530=CARTESIAN_POINT ( 'NONE',  ( -117.1020693116506379, -30.00000000000000000, -17.04080595179801705 ) ) ;
#7542=ORIENTED_EDGE ( 'NONE', *, *, #13036, .F. ) ;
#7549=AXIS2_PLACEMENT_3D ( 'NONE', #389, #6194, #11994 ) ;
#7590=CIRCLE ( 'NONE', #5780, 2.649999999999992806 ) ;
#7608=ADVANCED_FACE ( 'NONE', ( #16605 ), #12414, .F. ) ;
#7611=FACE_BOUND ( 'NONE', #17649, .T. ) ;
#7652=ORIENTED_EDGE ( 'NONE', *, *, #16675, .T. ) ;
#7687=LINE ( 'NONE', #12077, #4191 ) ;
#7735=DIRECTION ( 'NONE',  ( 2.220446049250313081E-16, 0.000000000000000000, -1.000000000000000000 ) ) ;
#7751=DIRECTION ( 'NONE',  ( 0.000000000000000000, 0.000000000000000000, 1.000000000000000000 ) ) ;
#7752=CARTESIAN_POINT ( 'NONE',  ( -56.50000000009000445, -34.99999999999999289, 2.650000000000374278 ) ) ;
#7756=VECTOR ( 'NONE', #13781, 1000.000000000000000 ) ;
#7794=EDGE_CURVE ( 'NONE', #9433, #114, #2979, .T. ) ;
#7833=CARTESIAN_POINT ( 'NONE',  ( -26.29305231718568336, -26.50000000000000000, -19.10302069950552095 ) ) ;
#7851=EDGE_CURVE ( 'NONE', #9159, #16839, #8688, .T. ) ;
#7859=DIRECTION ( 'NONE',  ( 2.220446049250313081E-16, 0.000000000000000000, 1.000000000000000000 ) ) ;
#7864=CIRCLE ( 'NONE', #10299, 2.649999999999992806 ) ;
#7915=AXIS2_PLACEMENT_3D ( 'NONE', #5160, #18215, #16789 ) ;
#7925=DIRECTION ( 'NONE',  ( 0.000000000000000000, 0.000000000000000000, 1.000000000000000000 ) ) ;
#7932=VERTEX_POINT ( 'NONE', #11737 ) ;
#7947=FACE_BOUND ( 'NONE', #4985, .T. ) ;
#7970=CIRCLE ( 'NONE', #18621, 2.649999999999985700 ) ;
#7994=DIRECTION ( 'NONE',  ( 0.000000000000000000, 0.000000000000000000, 1.000000000000000000 ) ) ;
#8004=( LENGTH_UNIT ( ) NAMED_UNIT ( * ) SI_UNIT ( .MILLI., .METRE. ) );
#8017=AXIS2_PLACEMENT_3D ( 'NONE', #12801, #14324, #9934 ) ;
#8024=EDGE_CURVE ( 'NONE', #139, #13167, #9527, .T. ) ;
#8035=CARTESIAN_POINT ( 'NONE',  ( -117.1020693116506379, -30.00000000000000000, -19.69080595179801207 ) ) ;
#8036=LINE ( 'NONE', #16527, #12474 ) ;
#8053=AXIS2_PLACEMENT_3D ( 'NONE', #12459, #18265, #5119 ) ;
#8075=ORIENTED_EDGE ( 'NONE', *, *, #578, .T. ) ;
#8120=CIRCLE ( 'NONE', #9639, 2.649999999999985700 ) ;
#8121=DIRECTION ( 'NONE',  ( 0.000000000000000000, 0.000000000000000000, 1.000000000000000000 ) ) ;
#8172=( LENGTH_UNIT ( ) NAMED_UNIT ( * ) SI_UNIT ( .MILLI., .METRE. ) );
#8174=CARTESIAN_POINT ( 'NONE',  ( 10.04305231718605285, -34.99999999999999289, -30.90933677959240811 ) ) ;
#8182=CIRCLE ( 'NONE', #6359, 2.649999999999995914 ) ;
#8191=EDGE_CURVE ( 'NONE', #10145, #15878, #8666, .T. ) ;
#8196=AXIS2_PLACEMENT_3D ( 'NONE', #4727, #1513, #9013 ) ;
#8205=DIRECTION ( 'NONE',  ( 0.000000000000000000, 0.000000000000000000, 1.000000000000000000 ) ) ;
#8216=ORIENTED_EDGE ( 'NONE', *, *, #1296, .T. ) ;
#8217=VERTEX_POINT ( 'NONE', #7240 ) ;
#8219=ORIENTED_EDGE ( 'NONE', *, *, #44, .F. ) ;
#8228=CARTESIAN_POINT ( 'NONE',  ( -79.64793068852898728, -30.00000000000000000, -34.51039329588755322 ) ) ;
#8235=ORIENTED_EDGE ( 'NONE', *, *, #372, .F. ) ;
#8260=ORIENTED_EDGE ( 'NONE', *, *, #14834, .F. ) ;
#8353=EDGE_LOOP ( 'NONE', ( #16636, #1593, #9713, #13305 ) ) ;
#8354=CARTESIAN_POINT ( 'NONE',  ( 32.50000000000000000, -34.99999999999999289, -2.649999999999631317 ) ) ;
#8369=EDGE_LOOP ( 'NONE', ( #9359, #17848, #13383, #5035 ) ) ;
#8436=ORIENTED_EDGE ( 'NONE', *, *, #917, .T. ) ;
#8459=CARTESIAN_POINT ( 'NONE',  ( -117.1020693116506379, -34.99999999999999289, -22.34080595179800355 ) ) ;
#8518=CARTESIAN_POINT ( 'NONE',  ( 10.04305231718605285, -34.99999999999999289, -33.55933677959240669 ) ) ;
#8524=EDGE_CURVE ( 'NONE', #9159, #16722, #7864, .T. ) ;
#8526=DIRECTION ( 'NONE',  ( 0.000000000000000000, -1.000000000000000000, 0.000000000000000000 ) ) ;
#8535=ORIENTED_EDGE ( 'NONE', *, *, #1328, .T. ) ;
#8541=ORIENTED_EDGE ( 'NONE', *, *, #4742, .T. ) ;
#8549=ORIENTED_EDGE ( 'NONE', *, *, #379, .F. ) ;
#8602=CARTESIAN_POINT ( 'NONE',  ( 10.04305231718579705, -34.99999999999999289, 33.55933677959249195 ) ) ;
#8613=VECTOR ( 'NONE', #14955, 1000.000000000000000 ) ;
#8656=FACE_OUTER_BOUND ( 'NONE', #11886, .T. ) ;
#8660=FACE_BOUND ( 'NONE', #1126, .T. ) ;
#8666=LINE ( 'NONE', #18588, #4509 ) ;
#8667=DIRECTION ( 'NONE',  ( -0.000000000000000000, -1.000000000000000000, -0.000000000000000000 ) ) ;
#8672=ORIENTED_EDGE ( 'NONE', *, *, #16492, .T. ) ;
#8688=LINE ( 'NONE', #4321, #10890 ) ;
#8694=VECTOR ( 'NONE', #10395, 1000.000000000000000 ) ;
#8752=FACE_OUTER_BOUND ( 'NONE', #4726, .T. ) ;
#8766=ADVANCED_FACE ( 'NONE', ( #14645 ), #15975, .F. ) ;
#8802=CARTESIAN_POINT ( 'NONE',  ( 10.04305231718579705, -34.99999999999999289, 30.90933677959249337 ) ) ;
#8818=LINE ( 'NONE', #1583, #6432 ) ;
#8825=ADVANCED_FACE ( 'NONE', ( #87 ), #1785, .F. ) ;
#8852=DIRECTION ( 'NONE',  ( 2.220446049250313081E-16, 0.000000000000000000, 1.000000000000000000 ) ) ;
#8876=AXIS2_PLACEMENT_3D ( 'NONE', #7232, #15906, #16184 ) ;
#8885=EDGE_CURVE ( 'NONE', #6727, #18475, #14887, .T. ) ;
#8902=VERTEX_POINT ( 'NONE', #9293 ) ;
#8912=ORIENTED_EDGE ( 'NONE', *, *, #15062, .F. ) ;
#8953=ORIENTED_EDGE ( 'NONE', *, *, #15623, .F. ) ;
#8955=ORIENTED_EDGE ( 'NONE', *, *, #18010, .T. ) ;
#9013=DIRECTION ( 'NONE',  ( 0.000000000000000000, 0.000000000000000000, 1.000000000000000000 ) ) ;
#9032=FACE_BOUND ( 'NONE', #12527, .T. ) ;
#9060=PRODUCT_DEFINITION_SHAPE ( 'NONE', 'NONE',  #14453 ) ;
#9071=ORIENTED_EDGE ( 'NONE', *, *, #17454, .T. ) ;
#9119=AXIS2_PLACEMENT_3D ( 'NONE', #9569, #15385, #17024 ) ;
#9122=AXIS2_PLACEMENT_3D ( 'NONE', #720, #12323, #16726 ) ;
#9126=CARTESIAN_POINT ( 'NONE',  ( 130.0000000000000000, -30.00000000000000000, 125.0000000000000000 ) ) ;
#9142=ORIENTED_EDGE ( 'NONE', *, *, #16328, .F. ) ;
#9145=DIRECTION ( 'NONE',  ( 0.000000000000000000, 0.000000000000000000, 1.000000000000000000 ) ) ;
#9153=EDGE_CURVE ( 'NONE', #10659, #5638, #7590, .T. ) ;
#9159=VERTEX_POINT ( 'NONE', #18306 ) ;
#9178=CARTESIAN_POINT ( 'NONE',  ( -290.0000000000001705, -34.99999999999999289, 125.0000000000000000 ) ) ;
#9185=CARTESIAN_POINT ( 'NONE',  ( -26.29305231718584324, -26.50000000000000000, 19.10302069950530779 ) ) ;
#9191=UNCERTAINTY_MEASURE_WITH_UNIT (LENGTH_MEASURE( 1.000000000000000082E-05 ), #8172, 'distance_accuracy_value', 'NONE');
#9198=ADVANCED_BREP_SHAPE_REPRESENTATION ( '', ( #10108, #8017 ), #3161 ) ;
#9202=AXIS2_PLACEMENT_3D ( 'NONE', #7488, #13309, #10257 ) ;
#9223=CARTESIAN_POINT ( 'NONE',  ( -90.00000000009001155, -30.00000000000000000, -1.301042606982605321E-15 ) ) ;
#9227=AXIS2_PLACEMENT_3D ( 'NONE', #4421, #8526, #10234 ) ;
#9236=EDGE_CURVE ( 'NONE', #5310, #16839, #13377, .T. ) ;
#9276=FACE_BOUND ( 'NONE', #9895, .T. ) ;
#9291=EDGE_CURVE ( 'NONE', #1567, #139, #8036, .T. ) ;
#9293=CARTESIAN_POINT ( 'NONE',  ( 10.04305231718605285, -30.00000000000000000, -28.25933677959240953 ) ) ;
#9302=DIRECTION ( 'NONE',  ( 0.000000000000000000, 1.000000000000000000, 0.000000000000000000 ) ) ;
#9320=CIRCLE ( 'NONE', #3559, 2.649999999999999467 ) ;
#9327=ADVANCED_FACE ( 'NONE', ( #4989 ), #13760, .F. ) ;
#9328=ADVANCED_FACE ( 'NONE', ( #818, #18138, #2144, #9276, #6622, #15009, #3584, #5090, #9556, #7947, #10619, #6340, #15371 ), #3763, .F. ) ;
#9355=ADVANCED_FACE ( 'NONE', ( #18044 ), #3388, .F. ) ;
#9357=DIRECTION ( 'NONE',  ( -0.000000000000000000, 1.000000000000000000, -0.000000000000000000 ) ) ;
#9359=ORIENTED_EDGE ( 'NONE', *, *, #3433, .F. ) ;
#9364=CARTESIAN_POINT ( 'NONE',  ( -79.64793068852927149, -30.00000000000000000, 34.51039329588763138 ) ) ;
#9426=CARTESIAN_POINT ( 'NONE',  ( 32.50000000000000000, -26.50000000000000000, 3.680389326632394941E-13 ) ) ;
#9433=VERTEX_POINT ( 'NONE', #8518 ) ;
#9434=AXIS2_PLACEMENT_3D ( 'NONE', #3175, #17563, #3089 ) ;
#9437=FILL_AREA_STYLE ('',( #398 ) ) ;
#9465=CARTESIAN_POINT ( 'NONE',  ( -26.29305231718584324, -34.99999999999999289, 19.10302069950530779 ) ) ;
#9472=DIRECTION ( 'NONE',  ( -0.000000000000000000, 1.000000000000000000, -0.000000000000000000 ) ) ;
#9514=AXIS2_PLACEMENT_3D ( 'NONE', #11047, #16870, #9624 ) ;
#9527=LINE ( 'NONE', #10762, #1470 ) ;
#9553=DIRECTION ( 'NONE',  ( -0.000000000000000000, -1.000000000000000000, -0.000000000000000000 ) ) ;
#9556=FACE_BOUND ( 'NONE', #10099, .T. ) ;
#9569=CARTESIAN_POINT ( 'NONE',  ( -117.1020693116508085, -30.00000000000000000, 19.69080595179778115 ) ) ;
#9579=CIRCLE ( 'NONE', #3320, 2.649999999999992806 ) ;
#9583=DIRECTION ( 'NONE',  ( -0.000000000000000000, 1.000000000000000000, -0.000000000000000000 ) ) ;
#9587=DIRECTION ( 'NONE',  ( -0.000000000000000000, -1.000000000000000000, -0.000000000000000000 ) ) ;
#9619=DIRECTION ( 'NONE',  ( -0.000000000000000000, -1.000000000000000000, -0.000000000000000000 ) ) ;
#9624=DIRECTION ( 'NONE',  ( 0.000000000000000000, 0.000000000000000000, 1.000000000000000000 ) ) ;
#9625=AXIS2_PLACEMENT_3D ( 'NONE', #1087, #18516, #5477 ) ;
#9629=AXIS2_PLACEMENT_3D ( 'NONE', #18094, #14965, #9145 ) ;
#9635=CARTESIAN_POINT ( 'NONE',  ( -26.29305231718584324, -26.50000000000000000, 16.45302069950530566 ) ) ;
#9639=AXIS2_PLACEMENT_3D ( 'NONE', #5122, #13790, #16269 ) ;
#9643=DIRECTION ( 'NONE',  ( 0.000000000000000000, 0.000000000000000000, -1.000000000000000000 ) ) ;
#9649=ORIENTED_EDGE ( 'NONE', *, *, #578, .F. ) ;
#9675=VECTOR ( 'NONE', #6290, 1000.000000000000000 ) ;
#9681=ADVANCED_FACE ( 'NONE', ( #13466 ), #409, .F. ) ;
#9713=ORIENTED_EDGE ( 'NONE', *, *, #10280, .F. ) ;
#9797=SURFACE_STYLE_USAGE ( .BOTH. , #15702 ) ;
#9801=CIRCLE ( 'NONE', #1584, 2.649999999999999467 ) ;
#9815=ORIENTED_EDGE ( 'NONE', *, *, #12482, .F. ) ;
#9841=EDGE_CURVE ( 'NONE', #17232, #139, #15345, .T. ) ;
#9849=EDGE_LOOP ( 'NONE', ( #8549, #3745, #18163, #7310 ) ) ;
#9856=CARTESIAN_POINT ( 'NONE',  ( -90.00000000009001155, -34.99999999999999289, 10.00000000000000711 ) ) ;
#9870=DIRECTION ( 'NONE',  ( 0.000000000000000000, 0.000000000000000000, 1.000000000000000000 ) ) ;
#9875=DIRECTION ( 'NONE',  ( 0.000000000000000000, 0.000000000000000000, 1.000000000000000000 ) ) ;
#9878=AXIS2_PLACEMENT_3D ( 'NONE', #10732, #9302, #5012 ) ;
#9895=EDGE_LOOP ( 'NONE', ( #1773, #18267 ) ) ;
#9908=FACE_OUTER_BOUND ( 'NONE', #1779, .T. ) ;
#9922=FACE_OUTER_BOUND ( 'NONE', #15875, .T. ) ;
#9934=DIRECTION ( 'NONE',  ( 1.000000000000000000, 0.000000000000000000, 0.000000000000000000 ) ) ;
#9942=ORIENTED_EDGE ( 'NONE', *, *, #2289, .F. ) ;
#9944=ADVANCED_FACE ( 'NONE', ( #4392 ), #7527, .F. ) ;
#9963=DIRECTION ( 'NONE',  ( 0.000000000000000000, 0.000000000000000000, 1.000000000000000000 ) ) ;
#9993=DIRECTION ( 'NONE',  ( -0.000000000000000000, 1.000000000000000000, -0.000000000000000000 ) ) ;
#9994=ORIENTED_EDGE ( 'NONE', *, *, #11796, .T. ) ;
#10001=CARTESIAN_POINT ( 'NONE',  ( -56.50000000009000445, -30.00000000000000000, -2.649999999999610889 ) ) ;
#10030=LINE ( 'NONE', #13081, #891 ) ;
#10034=DIRECTION ( 'NONE',  ( 0.000000000000000000, 0.000000000000000000, 1.000000000000000000 ) ) ;
#10099=EDGE_LOOP ( 'NONE', ( #14743, #6823 ) ) ;
#10108=MANIFOLD_SOLID_BREP ( 'M5 Clearance Hole4', #17734 ) ;
#10120=DIRECTION ( 'NONE',  ( -0.000000000000000000, -1.000000000000000000, -0.000000000000000000 ) ) ;
#10138=AXIS2_PLACEMENT_3D ( 'NONE', #9223, #1988, #2096 ) ;
#10145=VERTEX_POINT ( 'NONE', #8354 ) ;
#10154=EDGE_CURVE ( 'NONE', #18400, #6, #3982, .T. ) ;
#10167=CARTESIAN_POINT ( 'NONE',  ( -79.64793068852898728, -34.99999999999999289, -31.86039329588756530 ) ) ;
#10185=VERTEX_POINT ( 'NONE', #7102 ) ;
#10191=DIRECTION ( 'NONE',  ( -0.000000000000000000, 1.000000000000000000, -0.000000000000000000 ) ) ;
#10204=FACE_OUTER_BOUND ( 'NONE', #17983, .T. ) ;
#10213=EDGE_LOOP ( 'NONE', ( #13254, #15672, #3222, #2310 ) ) ;
#10234=DIRECTION ( 'NONE',  ( 0.000000000000000000, 0.000000000000000000, -1.000000000000000000 ) ) ;
#10257=DIRECTION ( 'NONE',  ( 0.000000000000000000, 0.000000000000000000, -1.000000000000000000 ) ) ;
#10264=CARTESIAN_POINT ( 'NONE',  ( 0.000000000000000000, -34.99999999999999289, 0.000000000000000000 ) ) ;
#10269=DIRECTION ( 'NONE',  ( 0.000000000000000000, 0.000000000000000000, 1.000000000000000000 ) ) ;
#10280=EDGE_CURVE ( 'NONE', #1567, #11247, #6146, .T. ) ;
#10281=DIRECTION ( 'NONE',  ( 0.000000000000000000, -1.000000000000000000, 0.000000000000000000 ) ) ;
#10284=FACE_BOUND ( 'NONE', #2404, .T. ) ;
#10294=EDGE_CURVE ( 'NONE', #7932, #15825, #8818, .T. ) ;
#10299=AXIS2_PLACEMENT_3D ( 'NONE', #10938, #15324, #3430 ) ;
#10359=DIRECTION ( 'NONE',  ( -0.000000000000000000, 1.000000000000000000, -0.000000000000000000 ) ) ;
#10380=CARTESIAN_POINT ( 'NONE',  ( -290.0000000000001137, -30.00000000000000000, -125.0000000000000000 ) ) ;
#10392=CIRCLE ( 'NONE', #16174, 2.649999999999995914 ) ;
#10395=DIRECTION ( 'NONE',  ( -0.000000000000000000, 1.000000000000000000, -0.000000000000000000 ) ) ;
#10410=DIRECTION ( 'NONE',  ( 0.000000000000000000, 0.000000000000000000, 1.000000000000000000 ) ) ;
#10479=VECTOR ( 'NONE', #14941, 1000.000000000000000 ) ;
#10481=EDGE_LOOP ( 'NONE', ( #766, #3900, #11914, #16255 ) ) ;
#10494=DIRECTION ( 'NONE',  ( 0.000000000000000000, 0.000000000000000000, 1.000000000000000000 ) ) ;
#10499=DIRECTION ( 'NONE',  ( 0.000000000000000000, 0.000000000000000000, -1.000000000000000000 ) ) ;
#10518=AXIS2_PLACEMENT_3D ( 'NONE', #11159, #14028, #17271 ) ;
#10543=CIRCLE ( 'NONE', #6901, 2.649999999999995914 ) ;
#10594=ORIENTED_EDGE ( 'NONE', *, *, #44, .T. ) ;
#10619=FACE_BOUND ( 'NONE', #1654, .T. ) ;
#10622=DIRECTION ( 'NONE',  ( 1.000000000000000000, 0.000000000000000000, 0.000000000000000000 ) ) ;
#10632=VERTEX_POINT ( 'NONE', #9856 ) ;
#10633=ORIENTED_EDGE ( 'NONE', *, *, #16346, .T. ) ;
#10659=VERTEX_POINT ( 'NONE', #4056 ) ;
#10691=PLANE ( 'NONE',  #11527 ) ;
#10731=DIRECTION ( 'NONE',  ( 0.000000000000000000, 0.000000000000000000, 1.000000000000000000 ) ) ;
#10732=CARTESIAN_POINT ( 'NONE',  ( -117.1020693116506379, -34.99999999999999289, -19.69080595179801207 ) ) ;
#10734=ORIENTED_EDGE ( 'NONE', *, *, #3433, .T. ) ;
#10747=EDGE_CURVE ( 'NONE', #16839, #5310, #5535, .T. ) ;
#10762=CARTESIAN_POINT ( 'NONE',  ( -290.0000000000001137, -30.00000000000000000, -125.0000000000000000 ) ) ;
#10772=ADVANCED_FACE ( 'NONE', ( #1476 ), #7451, .F. ) ;
#10775=LINE ( 'NONE', #17660, #17430 ) ;
#10777=ORIENTED_EDGE ( 'NONE', *, *, #6097, .F. ) ;
#10814=EDGE_CURVE ( 'NONE', #7932, #5476, #14605, .T. ) ;
#10875=DIRECTION ( 'NONE',  ( 0.000000000000000000, 1.000000000000000000, 0.000000000000000000 ) ) ;
#10890=VECTOR ( 'NONE', #2885, 1000.000000000000000 ) ;
#10917=ADVANCED_FACE ( 'NONE', ( #5065 ), #6597, .F. ) ;
#10920=LINE ( 'NONE', #4072, #2344 ) ;
#10933=VERTEX_POINT ( 'NONE', #3740 ) ;
#10938=CARTESIAN_POINT ( 'NONE',  ( -79.64793068852898728, -34.99999999999999289, -31.86039329588756530 ) ) ;
#10947=DIRECTION ( 'NONE',  ( 0.000000000000000000, 1.000000000000000000, 0.000000000000000000 ) ) ;
#10948=DIRECTION ( 'NONE',  ( 0.000000000000000000, 0.000000000000000000, 1.000000000000000000 ) ) ;
#10987=DIRECTION ( 'NONE',  ( -0.000000000000000000, 1.000000000000000000, -0.000000000000000000 ) ) ;
#10994=ADVANCED_FACE ( 'NONE', ( #9922 ), #2499, .F. ) ;
#11006=CIRCLE ( 'NONE', #8876, 2.649999999999985700 ) ;
#11047=CARTESIAN_POINT ( 'NONE',  ( -117.1020693116508085, -30.00000000000000000, 19.69080595179778115 ) ) ;
#11082=ORIENTED_EDGE ( 'NONE', *, *, #7256, .F. ) ;
#11131=ORIENTED_EDGE ( 'NONE', *, *, #71, .T. ) ;
#11141=ORIENTED_EDGE ( 'NONE', *, *, #14365, .T. ) ;
#11159=CARTESIAN_POINT ( 'NONE',  ( 10.04305231718579705, -26.50000000000000000, 30.90933677959249337 ) ) ;
#11167=DIRECTION ( 'NONE',  ( 0.000000000000000000, 1.000000000000000000, 0.000000000000000000 ) ) ;
#11240=DIRECTION ( 'NONE',  ( -0.000000000000000000, 1.000000000000000000, -0.000000000000000000 ) ) ;
#11247=VERTEX_POINT ( 'NONE', #4395 ) ;
#11344=EDGE_CURVE ( 'NONE', #15878, #11369, #9320, .T. ) ;
#11358=CARTESIAN_POINT ( 'NONE',  ( -56.50000000009000445, -34.99999999999999289, -2.649999999999610889 ) ) ;
#11369=VERTEX_POINT ( 'NONE', #15053 ) ;
#11370=EDGE_CURVE ( 'NONE', #12051, #3115, #5681, .T. ) ;
#11428=FACE_OUTER_BOUND ( 'NONE', #13148, .T. ) ;
#11431=CIRCLE ( 'NONE', #16588, 2.649999999999999467 ) ;
#11438=CIRCLE ( 'NONE', #13866, 2.649999999999992806 ) ;
#11465=VECTOR ( 'NONE', #13930, 1000.000000000000000 ) ;
#11481=EDGE_CURVE ( 'NONE', #12463, #17771, #2671, .T. ) ;
#11507=EDGE_LOOP ( 'NONE', ( #11528, #8953, #7652, #18540 ) ) ;
#11527=AXIS2_PLACEMENT_3D ( 'NONE', #1647, #14701, #7735 ) ;
#11528=ORIENTED_EDGE ( 'NONE', *, *, #11481, .F. ) ;
#11578=ADVANCED_FACE ( 'NONE', ( #14093 ), #6676, .F. ) ;
#11593=DIRECTION ( 'NONE',  ( -0.000000000000000000, 1.000000000000000000, -0.000000000000000000 ) ) ;
#11617=DIRECTION ( 'NONE',  ( 0.000000000000000000, 0.000000000000000000, 1.000000000000000000 ) ) ;
#11675=ADVANCED_FACE ( 'NONE', ( #8656 ), #7229, .F. ) ;
#11702=CARTESIAN_POINT ( 'NONE',  ( -56.50000000009000445, -30.00000000000000000, 2.650000000000367173 ) ) ;
#11711=CARTESIAN_POINT ( 'NONE',  ( -26.29305231718584324, -30.00000000000000000, 19.10302069950530779 ) ) ;
#11720=CIRCLE ( 'NONE', #17505, 20.00000000000000000 ) ;
#11737=CARTESIAN_POINT ( 'NONE',  ( -26.29305231718568336, -34.99999999999999289, -16.45302069950552237 ) ) ;
#11741=EDGE_CURVE ( 'NONE', #17771, #17376, #8120, .T. ) ;
#11750=EDGE_CURVE ( 'NONE', #13167, #16305, #5015, .T. ) ;
#11763=EDGE_LOOP ( 'NONE', ( #17929, #12945, #6553, #834 ) ) ;
#11796=EDGE_CURVE ( 'NONE', #833, #17767, #7687, .T. ) ;
#11809=FACE_BOUND ( 'NONE', #2339, .T. ) ;
#11847=FACE_OUTER_BOUND ( 'NONE', #13567, .T. ) ;
#11853=LINE ( 'NONE', #16235, #2679 ) ;
#11865=ORIENTED_EDGE ( 'NONE', *, *, #11750, .T. ) ;
#11886=EDGE_LOOP ( 'NONE', ( #6816, #5820, #6332, #12756 ) ) ;
#11888=FACE_OUTER_BOUND ( 'NONE', #8369, .T. ) ;
#11914=ORIENTED_EDGE ( 'NONE', *, *, #10154, .T. ) ;
#11919=( NAMED_UNIT ( * ) SI_UNIT ( $, .STERADIAN. ) SOLID_ANGLE_UNIT ( ) );
#11937=ORIENTED_EDGE ( 'NONE', *, *, #10280, .T. ) ;
#11940=CIRCLE ( 'NONE', #4948, 20.00000000000000000 ) ;
#11981=ORIENTED_EDGE ( 'NONE', *, *, #8885, .T. ) ;
#11994=DIRECTION ( 'NONE',  ( 0.000000000000000000, 0.000000000000000000, 1.000000000000000000 ) ) ;
#12009=EDGE_CURVE ( 'NONE', #18400, #3589, #11720, .T. ) ;
#12046=AXIS2_PLACEMENT_3D ( 'NONE', #15821, #2770, #14384 ) ;
#12051=VERTEX_POINT ( 'NONE', #14793 ) ;
#12075=CARTESIAN_POINT ( 'NONE',  ( -26.29305231718568336, -26.50000000000000000, -19.10302069950552095 ) ) ;
#12077=CARTESIAN_POINT ( 'NONE',  ( 10.04305231718579705, -26.50000000000000000, 33.55933677959249195 ) ) ;
#12087=CARTESIAN_POINT ( 'NONE',  ( -26.29305231718584324, -30.00000000000000000, 19.10302069950530779 ) ) ;
#12101=AXIS2_PLACEMENT_3D ( 'NONE', #600, #16501, #4690 ) ;
#12131=DIRECTION ( 'NONE',  ( -0.000000000000000000, 1.000000000000000000, -0.000000000000000000 ) ) ;
#12132=VECTOR ( 'NONE', #2102, 1000.000000000000000 ) ;
#12140=DIRECTION ( 'NONE',  ( 0.000000000000000000, 0.000000000000000000, 1.000000000000000000 ) ) ;
#12176=DIRECTION ( 'NONE',  ( -0.000000000000000000, 1.000000000000000000, -0.000000000000000000 ) ) ;
#12234=EDGE_CURVE ( 'NONE', #16305, #17232, #2034, .T. ) ;
#12253=CIRCLE ( 'NONE', #7385, 2.649999999999995914 ) ;
#12261=DIRECTION ( 'NONE',  ( -0.000000000000000000, 1.000000000000000000, -0.000000000000000000 ) ) ;
#12271=EDGE_LOOP ( 'NONE', ( #4929, #8955 ) ) ;
#12292=VERTEX_POINT ( 'NONE', #17176 ) ;
#12306=CARTESIAN_POINT ( 'NONE',  ( -79.64793068852927149, -34.99999999999999289, 31.86039329588764701 ) ) ;
#12323=DIRECTION ( 'NONE',  ( 0.000000000000000000, 1.000000000000000000, 0.000000000000000000 ) ) ;
#12341=CARTESIAN_POINT ( 'NONE',  ( -79.64793068852927149, -30.00000000000000000, 31.86039329588764701 ) ) ;
#12399=EDGE_CURVE ( 'NONE', #10145, #3496, #11431, .T. ) ;
#12414=PLANE ( 'NONE',  #3885 ) ;
#12459=CARTESIAN_POINT ( 'NONE',  ( 10.04305231718605285, -30.00000000000000000, -30.90933677959240811 ) ) ;
#12463=VERTEX_POINT ( 'NONE', #11358 ) ;
#12474=VECTOR ( 'NONE', #9472, 1000.000000000000000 ) ;
#12480=DIRECTION ( 'NONE',  ( -0.000000000000000000, 1.000000000000000000, -0.000000000000000000 ) ) ;
#12482=EDGE_CURVE ( 'NONE', #15024, #12292, #14878, .T. ) ;
#12505=DIRECTION ( 'NONE',  ( -1.000000000000000000, -0.000000000000000000, -0.000000000000000000 ) ) ;
#12525=EDGE_LOOP ( 'NONE', ( #15693, #10594, #7201, #4446 ) ) ;
#12527=EDGE_LOOP ( 'NONE', ( #8912, #13585 ) ) ;
#12543=DIRECTION ( 'NONE',  ( 0.000000000000000000, 1.000000000000000000, 0.000000000000000000 ) ) ;
#12550=EDGE_LOOP ( 'NONE', ( #10777, #7529 ) ) ;
#12572=DIRECTION ( 'NONE',  ( -0.000000000000000000, 1.000000000000000000, -0.000000000000000000 ) ) ;
#12619=ORIENTED_EDGE ( 'NONE', *, *, #14834, .T. ) ;
#12658=DIRECTION ( 'NONE',  ( -0.000000000000000000, -1.000000000000000000, -0.000000000000000000 ) ) ;
#12671=DIRECTION ( 'NONE',  ( -0.000000000000000000, 1.000000000000000000, -0.000000000000000000 ) ) ;
#12694=AXIS2_PLACEMENT_3D ( 'NONE', #11, #5807, #16182 ) ;
#12709=DIRECTION ( 'NONE',  ( 0.000000000000000000, 1.000000000000000000, 0.000000000000000000 ) ) ;
#12756=ORIENTED_EDGE ( 'NONE', *, *, #2827, .F. ) ;
#12760=EDGE_CURVE ( 'NONE', #2267, #16127, #15334, .T. ) ;
#12775=DIRECTION ( 'NONE',  ( -0.000000000000000000, 1.000000000000000000, -0.000000000000000000 ) ) ;
#12801=CARTESIAN_POINT ( 'NONE',  ( 0.000000000000000000, 0.000000000000000000, 0.000000000000000000 ) ) ;
#12819=ADVANCED_FACE ( 'NONE', ( #11428 ), #5446, .F. ) ;
#12876=EDGE_CURVE ( 'NONE', #10185, #421, #18442, .T. ) ;
#12899=DIRECTION ( 'NONE',  ( -0.000000000000000000, -1.000000000000000000, -0.000000000000000000 ) ) ;
#12900=ORIENTED_EDGE ( 'NONE', *, *, #12760, .F. ) ;
#12913=DIRECTION ( 'NONE',  ( 0.000000000000000000, 0.000000000000000000, 1.000000000000000000 ) ) ;
#12920=ADVANCED_FACE ( 'NONE', ( #8660, #10284, #11809, #3233, #14570, #5811, #15, #9032, #7611, #4563, #17348, #8752, #13147 ), #7415, .T. ) ;
#12923=DIRECTION ( 'NONE',  ( 0.000000000000000000, 0.000000000000000000, 1.000000000000000000 ) ) ;
#12945=ORIENTED_EDGE ( 'NONE', *, *, #2019, .T. ) ;
#12952=AXIS2_PLACEMENT_3D ( 'NONE', #13271, #227, #10494 ) ;
#12972=AXIS2_PLACEMENT_3D ( 'NONE', #7833, #3461, #7925 ) ;
#12988=AXIS2_PLACEMENT_3D ( 'NONE', #2678, #16100, #16188 ) ;
#12993=CARTESIAN_POINT ( 'NONE',  ( 10.04305231718605285, -34.99999999999999289, -30.90933677959240811 ) ) ;
#13005=CARTESIAN_POINT ( 'NONE',  ( -26.29305231718568336, -30.00000000000000000, -21.75302069950551953 ) ) ;
#13036=EDGE_CURVE ( 'NONE', #11369, #15878, #15707, .T. ) ;
#13056=VECTOR ( 'NONE', #14963, 1000.000000000000000 ) ;
#13058=ORIENTED_EDGE ( 'NONE', *, *, #1328, .F. ) ;
#13081=CARTESIAN_POINT ( 'NONE',  ( -90.00000000009001155, -29.99899999999999878, -10.00000000000001066 ) ) ;
#13087=ORIENTED_EDGE ( 'NONE', *, *, #15947, .T. ) ;
#13109=VERTEX_POINT ( 'NONE', #5019 ) ;
#13120=ORIENTED_EDGE ( 'NONE', *, *, #8191, .F. ) ;
#13147=FACE_BOUND ( 'NONE', #12271, .T. ) ;
#13148=EDGE_LOOP ( 'NONE', ( #312, #18180, #8436, #18242 ) ) ;
#13167=VERTEX_POINT ( 'NONE', #16554 ) ;
#13204=CARTESIAN_POINT ( 'NONE',  ( -290.0000000000001137, -34.99999999999999289, -125.0000000000000000 ) ) ;
#13254=ORIENTED_EDGE ( 'NONE', *, *, #7851, .F. ) ;
#13267=CARTESIAN_POINT ( 'NONE',  ( -290.0000000000001705, -34.99999999999999289, 125.0000000000000000 ) ) ;
#13271=CARTESIAN_POINT ( 'NONE',  ( -79.64793068852927149, -30.00000000000000000, 31.86039329588764701 ) ) ;
#13280=EDGE_LOOP ( 'NONE', ( #7112, #18602 ) ) ;
#13302=AXIS2_PLACEMENT_3D ( 'NONE', #12075, #17699, #13706 ) ;
#13305=ORIENTED_EDGE ( 'NONE', *, *, #9291, .T. ) ;
#13309=DIRECTION ( 'NONE',  ( 0.000000000000000000, -1.000000000000000000, 0.000000000000000000 ) ) ;
#13334=CYLINDRICAL_SURFACE ( 'NONE', #17603, 2.649999999999992806 ) ;
#13338=ORIENTED_EDGE ( 'NONE', *, *, #9153, .T. ) ;
#13345=CARTESIAN_POINT ( 'NONE',  ( 10.04305231718605285, -34.99999999999999289, -28.25933677959240953 ) ) ;
#13352=CARTESIAN_POINT ( 'NONE',  ( -290.0000000000001705, -34.99999999999999289, 125.0000000000000000 ) ) ;
#13377=CIRCLE ( 'NONE', #14897, 2.649999999999985700 ) ;
#13383=ORIENTED_EDGE ( 'NONE', *, *, #11741, .T. ) ;
#13432=ORIENTED_EDGE ( 'NONE', *, *, #71, .F. ) ;
#13448=CYLINDRICAL_SURFACE ( 'NONE', #7549, 2.649999999999995914 ) ;
#13466=FACE_OUTER_BOUND ( 'NONE', #3679, .T. ) ;
#13498=ORIENTED_EDGE ( 'NONE', *, *, #16346, .F. ) ;
#13533=CYLINDRICAL_SURFACE ( 'NONE', #7243, 2.649999999999992806 ) ;
#13544=EDGE_CURVE ( 'NONE', #14160, #1567, #18444, .T. ) ;
#13566=CARTESIAN_POINT ( 'NONE',  ( -290.0000000000001705, -34.99999999999999289, 125.0000000000000000 ) ) ;
#13567=EDGE_LOOP ( 'NONE', ( #18462, #8541, #11981, #13058 ) ) ;
#13584=AXIS2_PLACEMENT_3D ( 'NONE', #17617, #14661, #1525 ) ;
#13585=ORIENTED_EDGE ( 'NONE', *, *, #17302, .F. ) ;
#13604=ORIENTED_EDGE ( 'NONE', *, *, #7521, .F. ) ;
#13619=ORIENTED_EDGE ( 'NONE', *, *, #4687, .F. ) ;
#13634=CIRCLE ( 'NONE', #12101, 2.649999999999992806 ) ;
#13644=EDGE_CURVE ( 'NONE', #10933, #6918, #18633, .T. ) ;
#13698=AXIS2_PLACEMENT_3D ( 'NONE', #14788, #1743, #17741 ) ;
#13702=VECTOR ( 'NONE', #17169, 1000.000000000000000 ) ;
#13706=DIRECTION ( 'NONE',  ( 0.000000000000000000, 0.000000000000000000, 1.000000000000000000 ) ) ;
#13724=DIRECTION ( 'NONE',  ( 0.000000000000000000, 0.000000000000000000, 1.000000000000000000 ) ) ;
#13759=CYLINDRICAL_SURFACE ( 'NONE', #5948, 2.649999999999992806 ) ;
#13760=PLANE ( 'NONE',  #18253 ) ;
#13781=DIRECTION ( 'NONE',  ( 2.220446049250313081E-16, -0.000000000000000000, -1.000000000000000000 ) ) ;
#13790=DIRECTION ( 'NONE',  ( -0.000000000000000000, 1.000000000000000000, -0.000000000000000000 ) ) ;
#13803=MECHANICAL_DESIGN_GEOMETRIC_PRESENTATION_REPRESENTATION('',(#14714),#2246);
#13804=VERTEX_POINT ( 'NONE', #3197 ) ;
#13832=DIRECTION ( 'NONE',  ( 0.000000000000000000, 0.000000000000000000, 1.000000000000000000 ) ) ;
#13841=PRODUCT_DEFINITION_FORMATION_WITH_SPECIFIED_SOURCE ( 'ANY', '', #3293, .NOT_KNOWN. ) ;
#13849=ORIENTED_EDGE ( 'NONE', *, *, #9153, .F. ) ;
#13866=AXIS2_PLACEMENT_3D ( 'NONE', #18030, #18381, #5335 ) ;
#13878=VECTOR ( 'NONE', #16330, 1000.000000000000000 ) ;
#13888=VECTOR ( 'NONE', #12572, 1000.000000000000000 ) ;
#13930=DIRECTION ( 'NONE',  ( -0.000000000000000000, 1.000000000000000000, -0.000000000000000000 ) ) ;
#13977=ADVANCED_FACE ( 'NONE', ( #6804 ), #13759, .F. ) ;
#14028=DIRECTION ( 'NONE',  ( -0.000000000000000000, 1.000000000000000000, -0.000000000000000000 ) ) ;
#14086=AXIS2_PLACEMENT_3D ( 'NONE', #15185, #4605, #17838 ) ;
#14090=CARTESIAN_POINT ( 'NONE',  ( -79.64793068852927149, -30.00000000000000000, 29.21039329588765554 ) ) ;
#14093=FACE_OUTER_BOUND ( 'NONE', #2307, .T. ) ;
#14097=ORIENTED_EDGE ( 'NONE', *, *, #2954, .T. ) ;
#14139=UNCERTAINTY_MEASURE_WITH_UNIT (LENGTH_MEASURE( 1.000000000000000082E-05 ), #8004, 'distance_accuracy_value', 'NONE');
#14160=VERTEX_POINT ( 'NONE', #13267 ) ;
#14175=ORIENTED_EDGE ( 'NONE', *, *, #17564, .F. ) ;
#14180=DIRECTION ( 'NONE',  ( 0.000000000000000000, 0.000000000000000000, 1.000000000000000000 ) ) ;
#14256=CARTESIAN_POINT ( 'NONE',  ( -117.1020693116508085, -34.99999999999999289, 19.69080595179778115 ) ) ;
#14270=( NAMED_UNIT ( * ) PLANE_ANGLE_UNIT ( ) SI_UNIT ( $, .RADIAN. ) );
#14324=DIRECTION ( 'NONE',  ( 0.000000000000000000, 0.000000000000000000, 1.000000000000000000 ) ) ;
#14326=EDGE_LOOP ( 'NONE', ( #17213, #16045, #11131, #12900 ) ) ;
#14365=EDGE_CURVE ( 'NONE', #931, #6749, #5159, .T. ) ;
#14372=CARTESIAN_POINT ( 'NONE',  ( -117.1020693116506379, -30.00000000000000000, -19.69080595179801207 ) ) ;
#14384=DIRECTION ( 'NONE',  ( 0.000000000000000000, 0.000000000000000000, 1.000000000000000000 ) ) ;
#14397=LINE ( 'NONE', #5735, #6587 ) ;
#14406=DIRECTION ( 'NONE',  ( -0.000000000000000000, 1.000000000000000000, -0.000000000000000000 ) ) ;
#14437=CIRCLE ( 'NONE', #8053, 2.649999999999995914 ) ;
#14453=PRODUCT_DEFINITION ( 'UNKNOWN', '', #13841, #5787 ) ;
#14454=CARTESIAN_POINT ( 'NONE',  ( 0.000000000000000000, -34.99999999999999289, 0.000000000000000000 ) ) ;
#14475=EDGE_CURVE ( 'NONE', #3589, #2422, #14397, .T. ) ;
#14535=AXIS2_PLACEMENT_3D ( 'NONE', #12993, #12899, #10034 ) ;
#14569=AXIS2_PLACEMENT_3D ( 'NONE', #1051, #17424, #11617 ) ;
#14570=FACE_BOUND ( 'NONE', #348, .T. ) ;
#14605=CIRCLE ( 'NONE', #13698, 2.649999999999999467 ) ;
#14618=FACE_OUTER_BOUND ( 'NONE', #6129, .T. ) ;
#14645=FACE_OUTER_BOUND ( 'NONE', #10481, .T. ) ;
#14648=AXIS2_PLACEMENT_3D ( 'NONE', #14454, #17336, #1414 ) ;
#14659=CARTESIAN_POINT ( 'NONE',  ( -117.1020693116508085, -34.99999999999999289, 22.34080595179777262 ) ) ;
#14661=DIRECTION ( 'NONE',  ( 0.000000000000000000, 1.000000000000000000, 0.000000000000000000 ) ) ;
#14683=( LENGTH_UNIT ( ) NAMED_UNIT ( * ) SI_UNIT ( .MILLI., .METRE. ) );
#14701=DIRECTION ( 'NONE',  ( 1.000000000000000000, 0.000000000000000000, 2.220446049250313081E-16 ) ) ;
#14714=STYLED_ITEM ( 'NONE', ( #682 ), #9198 ) ;
#14743=ORIENTED_EDGE ( 'NONE', *, *, #2954, .F. ) ;
#14747=CARTESIAN_POINT ( 'NONE',  ( 32.50000000000000000, -30.00000000000000000, 3.680389326632394941E-13 ) ) ;
#14788=CARTESIAN_POINT ( 'NONE',  ( -26.29305231718568336, -34.99999999999999289, -19.10302069950552095 ) ) ;
#14793=CARTESIAN_POINT ( 'NONE',  ( -90.00000000009001155, -30.00000000000000000, -10.00000000000001066 ) ) ;
#14794=AXIS2_PLACEMENT_3D ( 'NONE', #3490, #257, #543 ) ;
#14812=CIRCLE ( 'NONE', #16038, 2.649999999999999467 ) ;
#14818=DIRECTION ( 'NONE',  ( -0.000000000000000000, 1.000000000000000000, -0.000000000000000000 ) ) ;
#14834=EDGE_CURVE ( 'NONE', #9433, #13109, #10920, .T. ) ;
#14839=EDGE_CURVE ( 'NONE', #6010, #15825, #14812, .T. ) ;
#14870=AXIS2_PLACEMENT_3D ( 'NONE', #9465, #9553, #12140 ) ;
#14878=LINE ( 'NONE', #4586, #8694 ) ;
#14887=CIRCLE ( 'NONE', #6671, 2.649999999999985700 ) ;
#14888=ORIENTED_EDGE ( 'NONE', *, *, #6542, .F. ) ;
#14897=AXIS2_PLACEMENT_3D ( 'NONE', #16703, #4887, #15460 ) ;
#14913=CIRCLE ( 'NONE', #9119, 2.649999999999985700 ) ;
#14941=DIRECTION ( 'NONE',  ( -0.000000000000000000, 1.000000000000000000, -0.000000000000000000 ) ) ;
#14955=DIRECTION ( 'NONE',  ( -0.000000000000000000, 1.000000000000000000, -0.000000000000000000 ) ) ;
#14963=DIRECTION ( 'NONE',  ( -0.000000000000000000, 1.000000000000000000, -0.000000000000000000 ) ) ;
#14965=DIRECTION ( 'NONE',  ( -0.000000000000000000, -1.000000000000000000, -0.000000000000000000 ) ) ;
#15009=FACE_BOUND ( 'NONE', #15476, .T. ) ;
#15017=DIRECTION ( 'NONE',  ( 0.000000000000000000, 0.000000000000000000, 1.000000000000000000 ) ) ;
#15024=VERTEX_POINT ( 'NONE', #16156 ) ;
#15053=CARTESIAN_POINT ( 'NONE',  ( 32.50000000000000000, -30.00000000000000000, 2.650000000000367617 ) ) ;
#15058=CARTESIAN_POINT ( 'NONE',  ( -117.1020693116508085, -30.00000000000000000, 22.34080595179777262 ) ) ;
#15062=EDGE_CURVE ( 'NONE', #3659, #13804, #16647, .T. ) ;
#15087=ORIENTED_EDGE ( 'NONE', *, *, #174, .T. ) ;
#15090=DIRECTION ( 'NONE',  ( -0.000000000000000000, 1.000000000000000000, -0.000000000000000000 ) ) ;
#15108=VERTEX_POINT ( 'NONE', #7752 ) ;
#15154=LINE ( 'NONE', #16771, #12132 ) ;
#15165=( NAMED_UNIT ( * ) SI_UNIT ( $, .STERADIAN. ) SOLID_ANGLE_UNIT ( ) );
#15185=CARTESIAN_POINT ( 'NONE',  ( -79.64793068852927149, -30.00000000000000000, 31.86039329588764701 ) ) ;
#15211=DIRECTION ( 'NONE',  ( 0.000000000000000000, 1.000000000000000000, 0.000000000000000000 ) ) ;
#15290=UNCERTAINTY_MEASURE_WITH_UNIT (LENGTH_MEASURE( 1.000000000000000082E-05 ), #14683, 'distance_accuracy_value', 'NONE');
#15309=EDGE_LOOP ( 'NONE', ( #15400, #1574 ) ) ;
#15324=DIRECTION ( 'NONE',  ( 0.000000000000000000, 1.000000000000000000, 0.000000000000000000 ) ) ;
#15334=LINE ( 'NONE', #15058, #3218 ) ;
#15345=LINE ( 'NONE', #2497, #13702 ) ;
#15365=DIRECTION ( 'NONE',  ( 0.000000000000000000, 0.000000000000000000, 1.000000000000000000 ) ) ;
#15369=VECTOR ( 'NONE', #12505, 1000.000000000000000 ) ;
#15371=FACE_BOUND ( 'NONE', #12550, .T. ) ;
#15385=DIRECTION ( 'NONE',  ( -0.000000000000000000, 1.000000000000000000, -0.000000000000000000 ) ) ;
#15398=CARTESIAN_POINT ( 'NONE',  ( -26.29305231718568336, -30.00000000000000000, -19.10302069950552095 ) ) ;
#15400=ORIENTED_EDGE ( 'NONE', *, *, #12876, .T. ) ;
#15407=DIRECTION ( 'NONE',  ( 0.000000000000000000, 0.000000000000000000, 1.000000000000000000 ) ) ;
#15460=DIRECTION ( 'NONE',  ( 0.000000000000000000, 0.000000000000000000, 1.000000000000000000 ) ) ;
#15476=EDGE_LOOP ( 'NONE', ( #13619, #9942 ) ) ;
#15557=ORIENTED_EDGE ( 'NONE', *, *, #174, .F. ) ;
#15587=CARTESIAN_POINT ( 'NONE',  ( -117.1020693116506379, -34.99999999999999289, -19.69080595179801207 ) ) ;
#15623=EDGE_CURVE ( 'NONE', #15108, #12463, #13634, .T. ) ;
#15632=CARTESIAN_POINT ( 'NONE',  ( -26.29305231718584324, -34.99999999999999289, 19.10302069950530779 ) ) ;
#15638=DIRECTION ( 'NONE',  ( -0.000000000000000000, 1.000000000000000000, -0.000000000000000000 ) ) ;
#15654=EDGE_CURVE ( 'NONE', #18475, #6727, #5729, .T. ) ;
#15658=ORIENTED_EDGE ( 'NONE', *, *, #14475, .T. ) ;
#15671=DIRECTION ( 'NONE',  ( -0.000000000000000000, 1.000000000000000000, -0.000000000000000000 ) ) ;
#15672=ORIENTED_EDGE ( 'NONE', *, *, #3966, .F. ) ;
#15680=AXIS2_PLACEMENT_3D ( 'NONE', #10167, #5966, #17596 ) ;
#15693=ORIENTED_EDGE ( 'NONE', *, *, #14365, .F. ) ;
#15702=SURFACE_SIDE_STYLE ('',( #7114 ) ) ;
#15707=CIRCLE ( 'NONE', #7477, 2.649999999999999467 ) ;
#15724=CARTESIAN_POINT ( 'NONE',  ( 10.04305231718579705, -26.50000000000000000, 30.90933677959249337 ) ) ;
#15727=CYLINDRICAL_SURFACE ( 'NONE', #12988, 10.00000000000000888 ) ;
#15730=AXIS2_PLACEMENT_3D ( 'NONE', #4736, #12176, #10731 ) ;
#15748=LINE ( 'NONE', #17178, #3945 ) ;
#15786=CIRCLE ( 'NONE', #14870, 2.649999999999999467 ) ;
#15808=CYLINDRICAL_SURFACE ( 'NONE', #14648, 20.00000000000000000 ) ;
#15821=CARTESIAN_POINT ( 'NONE',  ( -79.64793068852927149, -34.99999999999999289, 31.86039329588764701 ) ) ;
#15825=VERTEX_POINT ( 'NONE', #2299 ) ;
#15827=AXIS2_PLACEMENT_3D ( 'NONE', #1299, #15671, #12913 ) ;
#15829=AXIS2_PLACEMENT_3D ( 'NONE', #9185, #10987, #7751 ) ;
#15846=ORIENTED_EDGE ( 'NONE', *, *, #18325, .F. ) ;
#15875=EDGE_LOOP ( 'NONE', ( #6932, #3237, #9994, #6484 ) ) ;
#15878=VERTEX_POINT ( 'NONE', #16014 ) ;
#15894=AXIS2_PLACEMENT_3D ( 'NONE', #1159, #9619, #8205 ) ;
#15906=DIRECTION ( 'NONE',  ( -0.000000000000000000, 1.000000000000000000, -0.000000000000000000 ) ) ;
#15919=CIRCLE ( 'NONE', #10138, 10.00000000000000888 ) ;
#15947=EDGE_CURVE ( 'NONE', #10659, #3659, #16202, .T. ) ;
#15975=CYLINDRICAL_SURFACE ( 'NONE', #5767, 20.00000000000000000 ) ;
#15981=CARTESIAN_POINT ( 'NONE',  ( -290.0000000000001705, -30.00000000000000000, 125.0000000000000000 ) ) ;
#15983=ORIENTED_EDGE ( 'NONE', *, *, #10294, .T. ) ;
#16014=CARTESIAN_POINT ( 'NONE',  ( 32.50000000000000000, -30.00000000000000000, -2.649999999999631317 ) ) ;
#16015=EDGE_CURVE ( 'NONE', #11247, #13167, #15154, .T. ) ;
#16032=ORIENTED_EDGE ( 'NONE', *, *, #162, .F. ) ;
#16038=AXIS2_PLACEMENT_3D ( 'NONE', #15398, #12543, #9870 ) ;
#16042=CARTESIAN_POINT ( 'NONE',  ( -79.64793068852927149, -30.00000000000000000, 31.86039329588764701 ) ) ;
#16045=ORIENTED_EDGE ( 'NONE', *, *, #6542, .T. ) ;
#16093=CARTESIAN_POINT ( 'NONE',  ( -117.1020693116508085, -34.99999999999999289, 17.04080595179778967 ) ) ;
#16100=DIRECTION ( 'NONE',  ( -0.000000000000000000, -1.000000000000000000, -0.000000000000000000 ) ) ;
#16105=EDGE_CURVE ( 'NONE', #2267, #2260, #6041, .T. ) ;
#16127=VERTEX_POINT ( 'NONE', #2854 ) ;
#16139=FACE_OUTER_BOUND ( 'NONE', #5198, .T. ) ;
#16145=LINE ( 'NONE', #13566, #17290 ) ;
#16156=CARTESIAN_POINT ( 'NONE',  ( -26.29305231718584324, -34.99999999999999289, 21.75302069950530637 ) ) ;
#16174=AXIS2_PLACEMENT_3D ( 'NONE', #6841, #12658, #14180 ) ;
#16182=DIRECTION ( 'NONE',  ( 0.000000000000000000, 0.000000000000000000, 1.000000000000000000 ) ) ;
#16184=DIRECTION ( 'NONE',  ( 0.000000000000000000, 0.000000000000000000, 1.000000000000000000 ) ) ;
#16188=DIRECTION ( 'NONE',  ( 0.000000000000000000, 0.000000000000000000, -1.000000000000000000 ) ) ;
#16202=LINE ( 'NONE', #7530, #13056 ) ;
#16235=CARTESIAN_POINT ( 'NONE',  ( 10.04305231718605285, -26.50000000000000000, -28.25933677959240953 ) ) ;
#16255=ORIENTED_EDGE ( 'NONE', *, *, #18010, .F. ) ;
#16269=DIRECTION ( 'NONE',  ( 0.000000000000000000, 0.000000000000000000, 1.000000000000000000 ) ) ;
#16305=VERTEX_POINT ( 'NONE', #9126 ) ;
#16328=EDGE_CURVE ( 'NONE', #17285, #16305, #362, .T. ) ;
#16330=DIRECTION ( 'NONE',  ( -1.000000000000000000, -0.000000000000000000, -0.000000000000000000 ) ) ;
#16336=VECTOR ( 'NONE', #365, 1000.000000000000000 ) ;
#16346=EDGE_CURVE ( 'NONE', #8902, #13109, #14437, .T. ) ;
#16368=AXIS2_PLACEMENT_3D ( 'NONE', #17249, #10281, #5809 ) ;
#16387=LINE ( 'NONE', #3345, #8613 ) ;
#16419=CARTESIAN_POINT ( 'NONE',  ( -290.0000000000001137, -34.99999999999999289, -125.0000000000000000 ) ) ;
#16453=ORIENTED_EDGE ( 'NONE', *, *, #9841, .F. ) ;
#16462=FACE_OUTER_BOUND ( 'NONE', #14326, .T. ) ;
#16491=CARTESIAN_POINT ( 'NONE',  ( -79.64793068852927149, -30.00000000000000000, 29.21039329588766265 ) ) ;
#16492=EDGE_CURVE ( 'NONE', #5638, #10659, #18084, .T. ) ;
#16501=DIRECTION ( 'NONE',  ( 0.000000000000000000, 1.000000000000000000, 0.000000000000000000 ) ) ;
#16527=CARTESIAN_POINT ( 'NONE',  ( -290.0000000000001137, -34.99999999999999289, -125.0000000000000000 ) ) ;
#16535=CYLINDRICAL_SURFACE ( 'NONE', #14794, 10.00000000000000888 ) ;
#16551=DIRECTION ( 'NONE',  ( -0.000000000000000000, 1.000000000000000000, -0.000000000000000000 ) ) ;
#16552=CARTESIAN_POINT ( 'NONE',  ( -56.50000000009000445, -30.00000000000000000, 3.817814120399276590E-13 ) ) ;
#16554=CARTESIAN_POINT ( 'NONE',  ( 129.9999999999999432, -30.00000000000000000, -125.0000000000000000 ) ) ;
#16588=AXIS2_PLACEMENT_3D ( 'NONE', #2593, #10120, #17090 ) ;
#16605=FACE_OUTER_BOUND ( 'NONE', #8353, .T. ) ;
#16636=ORIENTED_EDGE ( 'NONE', *, *, #8024, .T. ) ;
#16647=CIRCLE ( 'NONE', #7523, 2.649999999999985700 ) ;
#16675=EDGE_CURVE ( 'NONE', #15108, #17376, #10775, .T. ) ;
#16703=CARTESIAN_POINT ( 'NONE',  ( -79.64793068852898728, -30.00000000000000000, -31.86039329588756530 ) ) ;
#16722=VERTEX_POINT ( 'NONE', #17745 ) ;
#16726=DIRECTION ( 'NONE',  ( 0.000000000000000000, -0.000000000000000000, 1.000000000000000000 ) ) ;
#16728=ORIENTED_EDGE ( 'NONE', *, *, #8024, .F. ) ;
#16746=ADVANCED_FACE ( 'NONE', ( #11847 ), #3465, .F. ) ;
#16763=( GEOMETRIC_REPRESENTATION_CONTEXT ( 3 ) GLOBAL_UNCERTAINTY_ASSIGNED_CONTEXT ( ( #9191 ) ) GLOBAL_UNIT_ASSIGNED_CONTEXT ( ( #8172, #14270, #5406 ) ) REPRESENTATION_CONTEXT ( 'NONE', 'WORKASPACE' ) );
#16769=EDGE_LOOP ( 'NONE', ( #15087, #801, #16939, #11937 ) ) ;
#16771=CARTESIAN_POINT ( 'NONE',  ( 129.9999999999999432, -34.99999999999999289, -125.0000000000000000 ) ) ;
#16784=EDGE_CURVE ( 'NONE', #6, #2422, #11940, .T. ) ;
#16789=DIRECTION ( 'NONE',  ( 0.000000000000000000, 0.000000000000000000, 1.000000000000000000 ) ) ;
#16821=APPLICATION_CONTEXT ( 'automotive_design' ) ;
#16833=AXIS2_PLACEMENT_3D ( 'NONE', #12087, #5024, #17903 ) ;
#16839=VERTEX_POINT ( 'NONE', #8228 ) ;
#16870=DIRECTION ( 'NONE',  ( -0.000000000000000000, 1.000000000000000000, -0.000000000000000000 ) ) ;
#16939=ORIENTED_EDGE ( 'NONE', *, *, #13544, .T. ) ;
#17001=CARTESIAN_POINT ( 'NONE',  ( -290.0000000000001137, -34.99999999999999289, -125.0000000000000000 ) ) ;
#17024=DIRECTION ( 'NONE',  ( 0.000000000000000000, 0.000000000000000000, 1.000000000000000000 ) ) ;
#17052=ORIENTED_EDGE ( 'NONE', *, *, #10747, .F. ) ;
#17079=CARTESIAN_POINT ( 'NONE',  ( 0.000000000000000000, -30.00000000000000000, 20.00000000000000000 ) ) ;
#17090=DIRECTION ( 'NONE',  ( 0.000000000000000000, 0.000000000000000000, 1.000000000000000000 ) ) ;
#17102=VECTOR ( 'NONE', #3156, 1000.000000000000000 ) ;
#17127=EDGE_LOOP ( 'NONE', ( #1405, #15658, #4006, #18244 ) ) ;
#17142=ORIENTED_EDGE ( 'NONE', *, *, #14839, .F. ) ;
#17155=DIRECTION ( 'NONE',  ( 0.000000000000000000, 0.000000000000000000, 1.000000000000000000 ) ) ;
#17161=EDGE_CURVE ( 'NONE', #5638, #13804, #6291, .T. ) ;
#17169=DIRECTION ( 'NONE',  ( 2.220446049250313081E-16, -0.000000000000000000, -1.000000000000000000 ) ) ;
#17176=CARTESIAN_POINT ( 'NONE',  ( -26.29305231718584324, -30.00000000000000000, 21.75302069950530637 ) ) ;
#17178=CARTESIAN_POINT ( 'NONE',  ( -117.1020693116508085, -30.00000000000000000, 17.04080595179778967 ) ) ;
#17213=ORIENTED_EDGE ( 'NONE', *, *, #4303, .F. ) ;
#17217=CYLINDRICAL_SURFACE ( 'NONE', #7524, 2.649999999999992806 ) ;
#17231=( NAMED_UNIT ( * ) PLANE_ANGLE_UNIT ( ) SI_UNIT ( $, .RADIAN. ) );
#17232=VERTEX_POINT ( 'NONE', #15981 ) ;
#17249=CARTESIAN_POINT ( 'NONE',  ( -90.00000000009001155, -34.99999999999999289, -1.301042606982605321E-15 ) ) ;
#17257=VECTOR ( 'NONE', #11240, 1000.000000000000000 ) ;
#17271=DIRECTION ( 'NONE',  ( 0.000000000000000000, 0.000000000000000000, 1.000000000000000000 ) ) ;
#17273=ADVANCED_FACE ( 'NONE', ( #4551 ), #15808, .F. ) ;
#17285=VERTEX_POINT ( 'NONE', #5609 ) ;
#17288=ORIENTED_EDGE ( 'NONE', *, *, #16328, .T. ) ;
#17290=VECTOR ( 'NONE', #15090, 1000.000000000000000 ) ;
#17302=EDGE_CURVE ( 'NONE', #13804, #3659, #7970, .T. ) ;
#17336=DIRECTION ( 'NONE',  ( -0.000000000000000000, 1.000000000000000000, -0.000000000000000000 ) ) ;
#17348=FACE_BOUND ( 'NONE', #5259, .T. ) ;
#17354=LINE ( 'NONE', #2868, #386 ) ;
#17356=VERTEX_POINT ( 'NONE', #5973 ) ;
#17376=VERTEX_POINT ( 'NONE', #11702 ) ;
#17424=DIRECTION ( 'NONE',  ( 0.000000000000000000, 1.000000000000000000, 0.000000000000000000 ) ) ;
#17430=VECTOR ( 'NONE', #9357, 1000.000000000000000 ) ;
#17454=EDGE_CURVE ( 'NONE', #5476, #7932, #4325, .T. ) ;
#17505=AXIS2_PLACEMENT_3D ( 'NONE', #4080, #4606, #10499 ) ;
#17557=EDGE_CURVE ( 'NONE', #12292, #6749, #9801, .T. ) ;
#17563=DIRECTION ( 'NONE',  ( -0.000000000000000000, 1.000000000000000000, -0.000000000000000000 ) ) ;
#17564=EDGE_CURVE ( 'NONE', #17376, #17771, #11006, .T. ) ;
#17596=DIRECTION ( 'NONE',  ( 0.000000000000000000, 0.000000000000000000, 1.000000000000000000 ) ) ;
#17603=AXIS2_PLACEMENT_3D ( 'NONE', #16552, #3509, #3230 ) ;
#17611=ORIENTED_EDGE ( 'NONE', *, *, #17302, .T. ) ;
#17616=DIRECTION ( 'NONE',  ( 0.000000000000000000, 1.000000000000000000, 0.000000000000000000 ) ) ;
#17617=CARTESIAN_POINT ( 'NONE',  ( 0.000000000000000000, -30.00000000000000000, 0.000000000000000000 ) ) ;
#17649=EDGE_LOOP ( 'NONE', ( #7026, #17052 ) ) ;
#17658=CARTESIAN_POINT ( 'NONE',  ( -79.64793068852898728, -30.00000000000000000, -31.86039329588756530 ) ) ;
#17660=CARTESIAN_POINT ( 'NONE',  ( -56.50000000009000445, -30.00000000000000000, 2.650000000000374278 ) ) ;
#17699=DIRECTION ( 'NONE',  ( -0.000000000000000000, 1.000000000000000000, -0.000000000000000000 ) ) ;
#17730=ORIENTED_EDGE ( 'NONE', *, *, #12009, .F. ) ;
#17734=CLOSED_SHELL ( 'NONE', ( #12819, #7290, #10917, #2079, #11578, #16746, #5028, #13977, #11675, #2494, #2846, #17273, #9328, #12920, #9327, #9944, #6215, #7608, #8766, #3513, #10772, #2099, #1919, #8825, #1447, #4762, #9681, #5417, #9355, #10994 ) ) ;
#17741=DIRECTION ( 'NONE',  ( 0.000000000000000000, 0.000000000000000000, 1.000000000000000000 ) ) ;
#17745=CARTESIAN_POINT ( 'NONE',  ( -79.64793068852898728, -34.99999999999999289, -29.21039329588757383 ) ) ;
#17767=VERTEX_POINT ( 'NONE', #460 ) ;
#17768=DIRECTION ( 'NONE',  ( -0.000000000000000000, -1.000000000000000000, -0.000000000000000000 ) ) ;
#17771=VERTEX_POINT ( 'NONE', #18174 ) ;
#17775=ORIENTED_EDGE ( 'NONE', *, *, #2996, .F. ) ;
#17783=ORIENTED_EDGE ( 'NONE', *, *, #13544, .F. ) ;
#17838=DIRECTION ( 'NONE',  ( 0.000000000000000000, 0.000000000000000000, 1.000000000000000000 ) ) ;
#17848=ORIENTED_EDGE ( 'NONE', *, *, #11481, .T. ) ;
#17872=FACE_OUTER_BOUND ( 'NONE', #9849, .T. ) ;
#17894=CARTESIAN_POINT ( 'NONE',  ( 2.449293598294706513E-15, -30.00000000000000000, -20.00000000000000000 ) ) ;
#17903=DIRECTION ( 'NONE',  ( 0.000000000000000000, 0.000000000000000000, 1.000000000000000000 ) ) ;
#17923=ORIENTED_EDGE ( 'NONE', *, *, #11370, .T. ) ;
#17929=ORIENTED_EDGE ( 'NONE', *, *, #10814, .T. ) ;
#17958=ORIENTED_EDGE ( 'NONE', *, *, #15623, .T. ) ;
#17975=MECHANICAL_DESIGN_GEOMETRIC_PRESENTATION_REPRESENTATION('',(#2773),#16763);
#17983=EDGE_LOOP ( 'NONE', ( #2888, #13849, #13087, #4639 ) ) ;
#18007=( NAMED_UNIT ( * ) PLANE_ANGLE_UNIT ( ) SI_UNIT ( $, .RADIAN. ) );
#18010=EDGE_CURVE ( 'NONE', #2422, #6, #18346, .T. ) ;
#18030=CARTESIAN_POINT ( 'NONE',  ( -56.50000000009000445, -34.99999999999999289, 3.817814120399276590E-13 ) ) ;
#18034=EDGE_LOOP ( 'NONE', ( #13498, #9649 ) ) ;
#18044=FACE_OUTER_BOUND ( 'NONE', #12525, .T. ) ;
#18072=CARTESIAN_POINT ( 'NONE',  ( 129.9999999999999432, -30.00000000000000000, -125.0000000000000000 ) ) ;
#18084=CIRCLE ( 'NONE', #9878, 2.649999999999992806 ) ;
#18094=CARTESIAN_POINT ( 'NONE',  ( -90.00000000009001155, -30.00000000000000000, -1.301042606982605321E-15 ) ) ;
#18106=VECTOR ( 'NONE', #11593, 1000.000000000000000 ) ;
#18138=FACE_BOUND ( 'NONE', #6590, .T. ) ;
#18149=AXIS2_PLACEMENT_3D ( 'NONE', #9426, #2188, #7994 ) ;
#18163=ORIENTED_EDGE ( 'NONE', *, *, #2289, .T. ) ;
#18168=VECTOR ( 'NONE', #12261, 1000.000000000000000 ) ;
#18174=CARTESIAN_POINT ( 'NONE',  ( -56.50000000009000445, -30.00000000000000000, -2.649999999999604228 ) ) ;
#18180=ORIENTED_EDGE ( 'NONE', *, *, #13644, .T. ) ;
#18212=ORIENTED_EDGE ( 'NONE', *, *, #7521, .T. ) ;
#18215=DIRECTION ( 'NONE',  ( -0.000000000000000000, 1.000000000000000000, -0.000000000000000000 ) ) ;
#18242=ORIENTED_EDGE ( 'NONE', *, *, #11796, .F. ) ;
#18244=ORIENTED_EDGE ( 'NONE', *, *, #10154, .F. ) ;
#18253=AXIS2_PLACEMENT_3D ( 'NONE', #533, #4815, #7859 ) ;
#18265=DIRECTION ( 'NONE',  ( 0.000000000000000000, 1.000000000000000000, 0.000000000000000000 ) ) ;
#18267=ORIENTED_EDGE ( 'NONE', *, *, #8524, .T. ) ;
#18285=DIRECTION ( 'NONE',  ( 0.000000000000000000, 0.000000000000000000, 1.000000000000000000 ) ) ;
#18306=CARTESIAN_POINT ( 'NONE',  ( -79.64793068852898728, -34.99999999999999289, -34.51039329588756033 ) ) ;
#18325=EDGE_CURVE ( 'NONE', #3589, #18400, #6173, .T. ) ;
#18346=CIRCLE ( 'NONE', #9202, 20.00000000000000000 ) ;
#18381=DIRECTION ( 'NONE',  ( 0.000000000000000000, 1.000000000000000000, 0.000000000000000000 ) ) ;
#18400=VERTEX_POINT ( 'NONE', #143 ) ;
#18442=CIRCLE ( 'NONE', #12046, 2.649999999999992806 ) ;
#18444=LINE ( 'NONE', #842, #7756 ) ;
#18447=CARTESIAN_POINT ( 'NONE',  ( 0.000000000000000000, -34.99999999999999289, 20.00000000000000000 ) ) ;
#18453=CARTESIAN_POINT ( 'NONE',  ( -26.29305231718568336, -34.99999999999999289, -21.75302069950551953 ) ) ;
#18455=ORIENTED_EDGE ( 'NONE', *, *, #9291, .F. ) ;
#18462=ORIENTED_EDGE ( 'NONE', *, *, #6302, .F. ) ;
#18475=VERTEX_POINT ( 'NONE', #9364 ) ;
#18479=CARTESIAN_POINT ( 'NONE',  ( 32.50000000000000000, -26.50000000000000000, 3.680389326632394941E-13 ) ) ;
#18516=DIRECTION ( 'NONE',  ( 0.000000000000000000, -1.000000000000000000, 0.000000000000000000 ) ) ;
#18538=ORIENTED_EDGE ( 'NONE', *, *, #7794, .T. ) ;
#18540=ORIENTED_EDGE ( 'NONE', *, *, #17564, .T. ) ;
#18587=CARTESIAN_POINT ( 'NONE',  ( 32.50000000000000000, -34.99999999999999289, 2.650000000000367617 ) ) ;
#18588=CARTESIAN_POINT ( 'NONE',  ( 32.50000000000000000, -26.50000000000000000, -2.649999999999631317 ) ) ;
#18602=ORIENTED_EDGE ( 'NONE', *, *, #8885, .F. ) ;
#18621=AXIS2_PLACEMENT_3D ( 'NONE', #14372, #9993, #10269 ) ;
#18626=EDGE_LOOP ( 'NONE', ( #13338, #8672 ) ) ;
#18633=LINE ( 'NONE', #3019, #18106 ) ;
#18637=DIRECTION ( 'NONE',  ( -0.000000000000000000, 1.000000000000000000, -0.000000000000000000 ) ) ;
#18649=SHAPE_REPRESENTATION_RELATIONSHIP ( 'NONE' , 'NONE' ,  #18682, #9198 ) ;
#18682=SHAPE_REPRESENTATION ( 'base plate', ( #8017 ), #3161 ) ;
#18736=AXIS2_PLACEMENT_3D ( 'NONE', #14256, #2626, #9963 ) ;
#18743=EDGE_LOOP ( 'NONE', ( #8216, #12619, #8075, #13604 ) ) ;
#18771=LINE ( 'NONE', #6092, #6163 ) ;
#18849=COLOUR_RGB('Dark Blue',0.08,0.2,0.34);
#18850=FILL_AREA_STYLE_COLOUR('',#18849);
#18851=FILL_AREA_STYLE('',(#18850));
#18852=SURFACE_STYLE_FILL_AREA(#18851);
#18853=SURFACE_SIDE_STYLE('',(#18852));
#18854=SURFACE_STYLE_USAGE(.BOTH.,#18853);
#18855=PRESENTATION_STYLE_ASSIGNMENT((#18854));
ENDSEC;
END-ISO-10303-21;
